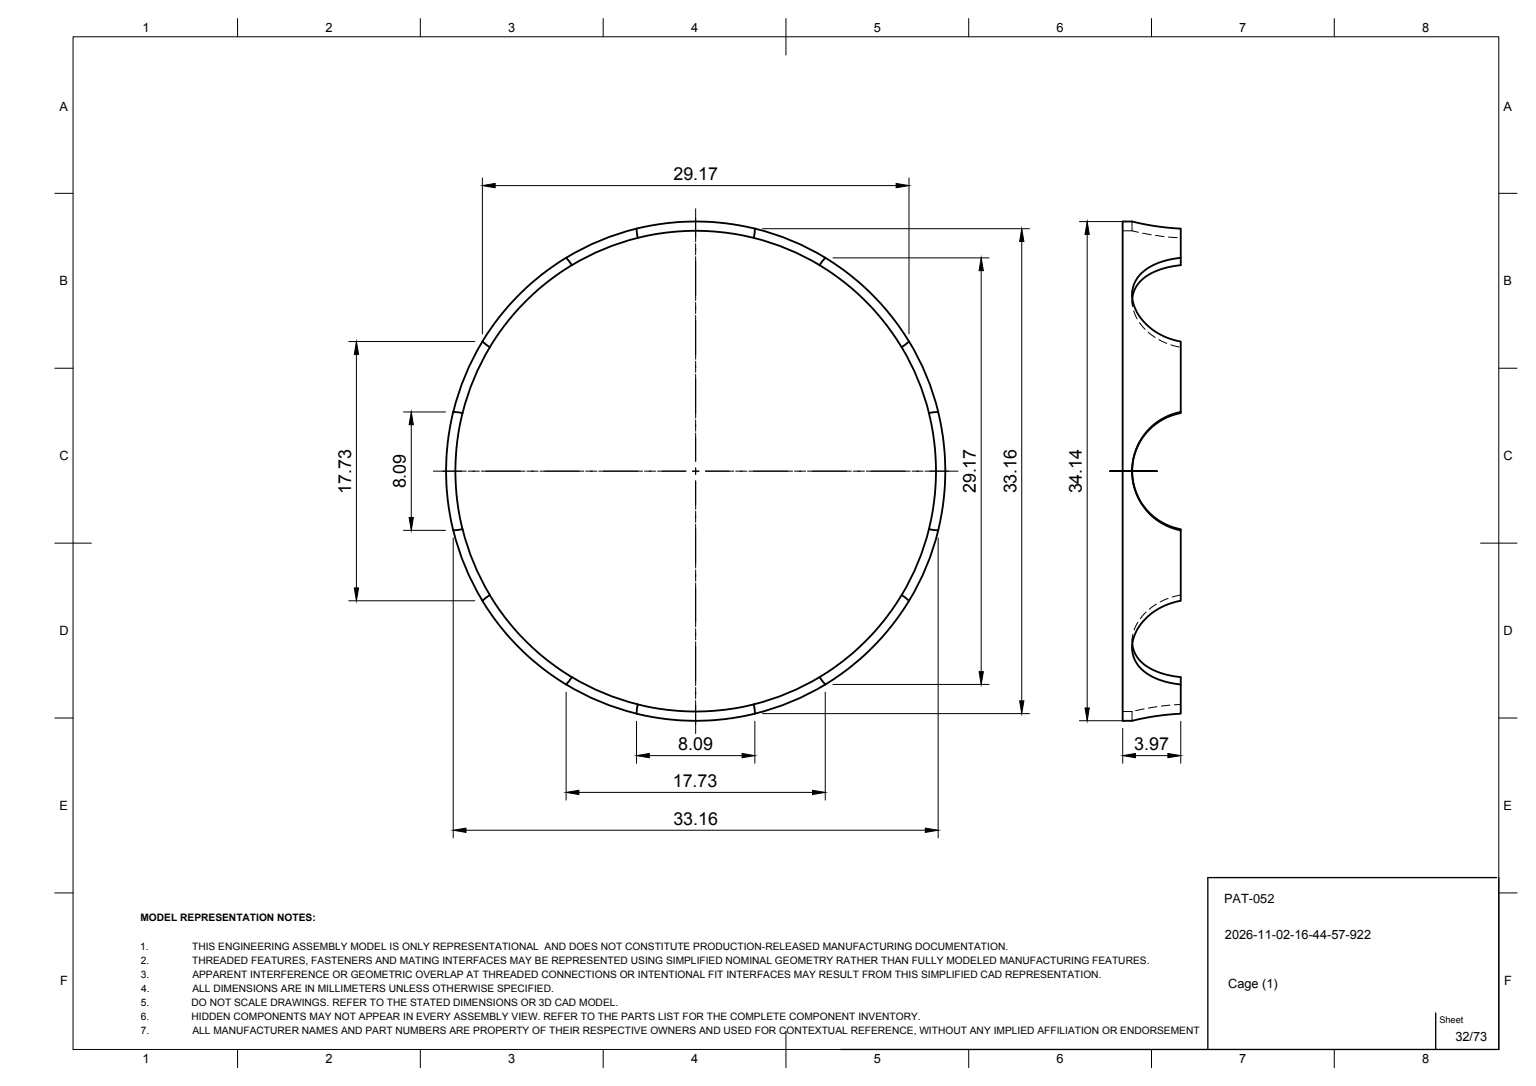
ISO-10303-21;
HEADER;
/* Generated by software containing ST-Developer
 * from STEP Tools, Inc. (www.steptools.com) 
 */

FILE_DESCRIPTION(
/* description */ ('Hand-crank gear train demonstrator'),
/* implementation_level */ '2;1');

FILE_NAME(
/* name */ 'Cage (1).step',
/* time_stamp */ '2026-10-28T03:22:13-07:00',
/* author */ (''),
/* organization */ (''),
/* preprocessor_version */ 'ST-DEVELOPER v20.2',
/* originating_system */ 'Autodesk Translation Framework v15.17.0.0',
/* authorisation */ '');

FILE_SCHEMA (('AUTOMOTIVE_DESIGN { 1 0 10303 214 3 1 1 }'));
ENDSEC;

DATA;
#10=MECHANICAL_DESIGN_GEOMETRIC_PRESENTATION_REPRESENTATION('',(#1222),#62758);
#873=B_SPLINE_CURVE_WITH_KNOTS('',3,(#24613,#24614,#24615,#24616,#24617,
#24618,#24619,#24620,#24621,#24622,#24623,#24624,#24625,#24626,#24627,#24628,
#24629,#24630,#24631,#24632,#24633,#24634),.UNSPECIFIED.,.F.,.F.,(4,2,2,
2,2,2,2,2,2,2,4),(0.0789094028588958,0.210573405340968,0.315860108011452,
0.421146810681936,0.522142632548711,0.623138454415485,0.72413427628226,
0.825130098149035,0.930416800819519,1.03570350349,1.16736750597208),
 .UNSPECIFIED.);
#874=B_SPLINE_CURVE_WITH_KNOTS('',3,(#24638,#24639,#24640,#24641,#24642,
#24643,#24644,#24645,#24646,#24647,#24648,#24649,#24650,#24651,#24652,#24653,
#24654,#24655,#24656,#24657,#24658,#24659),.UNSPECIFIED.,.F.,.F.,(4,2,2,
2,2,2,2,2,2,2,4),(0.0774793363974613,0.142088896491891,0.284177792983782,
0.411119756996526,0.514392970548519,0.617666184100513,0.720939397652506,
0.8242126112045,0.951154575217244,1.09324347170913,1.15785303180356),
 .UNSPECIFIED.);
#875=B_SPLINE_CURVE_WITH_KNOTS('',3,(#24665,#24666,#24667,#24668,#24669,
#24670,#24671,#24672,#24673,#24674,#24675,#24676,#24677,#24678,#24679,#24680,
#24681,#24682,#24683,#24684,#24685,#24686),.UNSPECIFIED.,.F.,.F.,(4,2,2,
2,2,2,2,2,2,2,4),(0.0774793363974613,0.142088896491891,0.284177792983782,
0.411119756996525,0.514392970548519,0.617666184100513,0.720939397652506,
0.8242126112045,0.951154575217243,1.09324347170913,1.15785303180356),
 .UNSPECIFIED.);
#876=B_SPLINE_CURVE_WITH_KNOTS('',3,(#24690,#24691,#24692,#24693,#24694,
#24695,#24696,#24697,#24698,#24699,#24700,#24701,#24702,#24703,#24704,#24705,
#24706,#24707,#24708,#24709,#24710,#24711),.UNSPECIFIED.,.F.,.F.,(4,2,2,
2,2,2,2,2,2,2,4),(0.0774793363974614,0.142088896491891,0.284177792983781,
0.411119756996525,0.514392970548519,0.617666184100512,0.720939397652506,
0.824212611204499,0.951154575217243,1.09324347170913,1.15785303180356),
 .UNSPECIFIED.);
#877=B_SPLINE_CURVE_WITH_KNOTS('',3,(#24715,#24716,#24717,#24718,#24719,
#24720,#24721,#24722,#24723,#24724,#24725,#24726),.UNSPECIFIED.,.F.,.F.,
(4,2,2,2,2,4),(0.0774793363974613,0.142088896491891,0.284177792983781,0.411119756996525,
0.514392970548519,0.617666184100512),.UNSPECIFIED.);
#878=B_SPLINE_CURVE_WITH_KNOTS('',3,(#24731,#24732,#24733,#24734,#24735,
#24736,#24737,#24738,#24739,#24740,#24741,#24742),.UNSPECIFIED.,.F.,.F.,
(4,2,2,2,2,4),(0.617666184100512,0.720939397652506,0.824212611204499,0.951154575217243,
1.09324347170913,1.15785303180356),.UNSPECIFIED.);
#879=B_SPLINE_CURVE_WITH_KNOTS('',3,(#24746,#24747,#24748,#24749,#24750,
#24751,#24752,#24753,#24754,#24755,#24756,#24757,#24758,#24759,#24760,#24761,
#24762,#24763,#24764,#24765,#24766,#24767),.UNSPECIFIED.,.F.,.F.,(4,2,2,
2,2,2,2,2,2,2,4),(0.0774793363974613,0.142088896491891,0.284177792983782,
0.411119756996526,0.514392970548519,0.617666184100513,0.720939397652507,
0.8242126112045,0.951154575217245,1.09324347170914,1.15785303180356),
 .UNSPECIFIED.);
#880=B_SPLINE_CURVE_WITH_KNOTS('',3,(#24771,#24772,#24773,#24774,#24775,
#24776,#24777,#24778,#24779,#24780,#24781,#24782,#24783,#24784,#24785,#24786,
#24787,#24788,#24789,#24790,#24791,#24792),.UNSPECIFIED.,.F.,.F.,(4,2,2,
2,2,2,2,2,2,2,4),(0.0774793363974613,0.142088896491891,0.284177792983782,
0.411119756996526,0.514392970548519,0.617666184100513,0.720939397652506,
0.824212611204499,0.951154575217243,1.09324347170913,1.15785303180356),
 .UNSPECIFIED.);
#881=B_SPLINE_CURVE_WITH_KNOTS('',3,(#24796,#24797,#24798,#24799,#24800,
#24801,#24802,#24803,#24804,#24805,#24806,#24807,#24808,#24809,#24810,#24811,
#24812,#24813,#24814,#24815,#24816,#24817),.UNSPECIFIED.,.F.,.F.,(4,2,2,
2,2,2,2,2,2,2,4),(0.0774793363974613,0.142088896491891,0.284177792983782,
0.411119756996526,0.514392970548519,0.617666184100513,0.720939397652506,
0.8242126112045,0.951154575217244,1.09324347170913,1.15785303180356),
 .UNSPECIFIED.);
#882=B_SPLINE_CURVE_WITH_KNOTS('',3,(#24821,#24822,#24823,#24824,#24825,
#24826,#24827,#24828,#24829,#24830,#24831,#24832,#24833,#24834,#24835,#24836,
#24837,#24838,#24839,#24840,#24841,#24842),.UNSPECIFIED.,.F.,.F.,(4,2,2,
2,2,2,2,2,2,2,4),(0.0774793363974613,0.142088896491891,0.284177792983782,
0.411119756996526,0.514392970548519,0.617666184100513,0.720939397652506,
0.8242126112045,0.951154575217243,1.09324347170913,1.15785303180356),
 .UNSPECIFIED.);
#883=B_SPLINE_CURVE_WITH_KNOTS('',3,(#24850,#24851,#24852,#24853,#24854,
#24855,#24856,#24857,#24858,#24859,#24860,#24861,#24862,#24863,#24864,#24865,
#24866,#24867,#24868,#24869,#24870,#24871),.UNSPECIFIED.,.F.,.F.,(4,2,2,
2,2,2,2,2,2,2,4),(0.0789094028588958,0.210573405340968,0.315860108011452,
0.421146810681936,0.522142632548711,0.623138454415485,0.72413427628226,
0.825130098149035,0.930416800819519,1.03570350349,1.16736750597208),
 .UNSPECIFIED.);
#884=B_SPLINE_CURVE_WITH_KNOTS('',3,(#24879,#24880,#24881,#24882,#24883,
#24884,#24885,#24886,#24887,#24888,#24889,#24890,#24891,#24892,#24893,#24894,
#24895,#24896,#24897,#24898,#24899,#24900),.UNSPECIFIED.,.F.,.F.,(4,2,2,
2,2,2,2,2,2,2,4),(0.0789094028588958,0.210573405340969,0.315860108011453,
0.421146810681937,0.522142632548712,0.623138454415486,0.724134276282261,
0.825130098149035,0.930416800819519,1.03570350349,1.16736750597208),
 .UNSPECIFIED.);
#885=B_SPLINE_CURVE_WITH_KNOTS('',3,(#24909,#24910,#24911,#24912,#24913,
#24914,#24915,#24916,#24917,#24918,#24919,#24920),.UNSPECIFIED.,.F.,.F.,
(4,2,2,2,2,4),(0.0789094028588958,0.210573405340968,0.315860108011452,0.421146810681937,
0.522142632548711,0.623138454415486),.UNSPECIFIED.);
#886=B_SPLINE_CURVE_WITH_KNOTS('',3,(#24922,#24923,#24924,#24925,#24926,
#24927,#24928,#24929,#24930,#24931,#24932,#24933),.UNSPECIFIED.,.F.,.F.,
(4,2,2,2,2,4),(0.623138454415486,0.72413427628226,0.825130098149035,0.930416800819519,
1.03570350349,1.16736750597208),.UNSPECIFIED.);
#887=B_SPLINE_CURVE_WITH_KNOTS('',3,(#24940,#24941,#24942,#24943,#24944,
#24945,#24946,#24947,#24948,#24949,#24950,#24951,#24952,#24953,#24954,#24955,
#24956,#24957,#24958,#24959,#24960,#24961),.UNSPECIFIED.,.F.,.F.,(4,2,2,
2,2,2,2,2,2,2,4),(0.0789094028588958,0.210573405340968,0.315860108011452,
0.421146810681936,0.522142632548711,0.623138454415486,0.72413427628226,
0.825130098149035,0.930416800819519,1.03570350349,1.16736750597208),
 .UNSPECIFIED.);
#888=B_SPLINE_CURVE_WITH_KNOTS('',3,(#24969,#24970,#24971,#24972,#24973,
#24974,#24975,#24976,#24977,#24978,#24979,#24980,#24981,#24982,#24983,#24984,
#24985,#24986,#24987,#24988,#24989,#24990),.UNSPECIFIED.,.F.,.F.,(4,2,2,
2,2,2,2,2,2,2,4),(0.0789094028588957,0.210573405340968,0.315860108011452,
0.421146810681936,0.522142632548711,0.623138454415485,0.72413427628226,
0.825130098149035,0.930416800819519,1.03570350349,1.16736750597207),
 .UNSPECIFIED.);
#889=B_SPLINE_CURVE_WITH_KNOTS('',3,(#24998,#24999,#25000,#25001,#25002,
#25003,#25004,#25005,#25006,#25007,#25008,#25009,#25010,#25011,#25012,#25013,
#25014,#25015,#25016,#25017,#25018,#25019),.UNSPECIFIED.,.F.,.F.,(4,2,2,
2,2,2,2,2,2,2,4),(0.0789094028588958,0.210573405340968,0.315860108011452,
0.421146810681936,0.522142632548711,0.623138454415486,0.72413427628226,
0.825130098149035,0.930416800819519,1.03570350349,1.16736750597208),
 .UNSPECIFIED.);
#890=B_SPLINE_CURVE_WITH_KNOTS('',3,(#25028,#25029,#25030,#25031,#25032,
#25033,#25034,#25035,#25036,#25037,#25038,#25039,#25040,#25041,#25042,#25043,
#25044,#25045,#25046,#25047,#25048,#25049),.UNSPECIFIED.,.F.,.F.,(4,2,2,
2,2,2,2,2,2,2,4),(0.0789094028588958,0.210573405340968,0.315860108011452,
0.421146810681936,0.522142632548711,0.623138454415485,0.72413427628226,
0.825130098149035,0.930416800819519,1.03570350349,1.16736750597208),
 .UNSPECIFIED.);
#1013=SPHERICAL_SURFACE('',#17671,0.412776);
#1014=SPHERICAL_SURFACE('',#17687,0.412776);
#1015=SPHERICAL_SURFACE('',#17692,0.412776);
#1016=SPHERICAL_SURFACE('',#17697,0.412776);
#1017=SPHERICAL_SURFACE('',#17702,0.412776);
#1018=SPHERICAL_SURFACE('',#17707,0.412776);
#1019=SPHERICAL_SURFACE('',#17712,0.412776);
#1020=SPHERICAL_SURFACE('',#17720,0.412776);
#1080=SHAPE_REPRESENTATION_RELATIONSHIP('SRR','None',#63054,#1144);
#1144=ADVANCED_BREP_SHAPE_REPRESENTATION('',(#1300),#62708);
#1222=STYLED_ITEM('',(#63462),#1300);
#1300=MANIFOLD_SOLID_BREP('Continuous crown cage',#16403);
#1500=FACE_BOUND('',#3445,.T.);
#1702=PLANE('',#17684);
#1703=PLANE('',#17689);
#1704=PLANE('',#17694);
#1705=PLANE('',#17699);
#1706=PLANE('',#17704);
#1707=PLANE('',#17709);
#1708=PLANE('',#17718);
#1709=PLANE('',#17722);
#1710=PLANE('',#17723);
#2333=FACE_OUTER_BOUND('',#3427,.T.);
#2334=FACE_OUTER_BOUND('',#3428,.T.);
#2335=FACE_OUTER_BOUND('',#3429,.T.);
#2336=FACE_OUTER_BOUND('',#3430,.T.);
#2337=FACE_OUTER_BOUND('',#3431,.T.);
#2338=FACE_OUTER_BOUND('',#3432,.T.);
#2339=FACE_OUTER_BOUND('',#3433,.T.);
#2340=FACE_OUTER_BOUND('',#3434,.T.);
#2341=FACE_OUTER_BOUND('',#3435,.T.);
#2342=FACE_OUTER_BOUND('',#3436,.T.);
#2343=FACE_OUTER_BOUND('',#3437,.T.);
#2344=FACE_OUTER_BOUND('',#3438,.T.);
#2345=FACE_OUTER_BOUND('',#3439,.T.);
#2346=FACE_OUTER_BOUND('',#3440,.T.);
#2347=FACE_OUTER_BOUND('',#3441,.T.);
#2348=FACE_OUTER_BOUND('',#3442,.T.);
#2349=FACE_OUTER_BOUND('',#3443,.T.);
#2350=FACE_OUTER_BOUND('',#3444,.T.);
#2351=FACE_OUTER_BOUND('',#3446,.T.);
#3427=EDGE_LOOP('',(#11737,#11738,#11739,#11740));
#3428=EDGE_LOOP('',(#11741,#11742,#11743,#11744,#11745,#11746,#11747,#11748,
#11749,#11750,#11751,#11752,#11753,#11754,#11755,#11756,#11757,#11758,#11759,
#11760));
#3429=EDGE_LOOP('',(#11761,#11762,#11763,#11764));
#3430=EDGE_LOOP('',(#11765,#11766,#11767,#11768));
#3431=EDGE_LOOP('',(#11769,#11770,#11771,#11772));
#3432=EDGE_LOOP('',(#11773,#11774,#11775,#11776));
#3433=EDGE_LOOP('',(#11777,#11778,#11779,#11780));
#3434=EDGE_LOOP('',(#11781,#11782,#11783,#11784,#11785,#11786));
#3435=EDGE_LOOP('',(#11787,#11788,#11789,#11790));
#3436=EDGE_LOOP('',(#11791,#11792,#11793,#11794));
#3437=EDGE_LOOP('',(#11795,#11796,#11797,#11798));
#3438=EDGE_LOOP('',(#11799,#11800,#11801,#11802));
#3439=EDGE_LOOP('',(#11803,#11804,#11805,#11806));
#3440=EDGE_LOOP('',(#11807,#11808,#11809,#11810));
#3441=EDGE_LOOP('',(#11811,#11812,#11813,#11814,#11815,#11816,#11817,#11818,
#11819,#11820,#11821,#11822,#11823,#11824,#11825,#11826,#11827,#11828,#11829,
#11830));
#3442=EDGE_LOOP('',(#11831,#11832,#11833,#11834));
#3443=EDGE_LOOP('',(#11835,#11836,#11837,#11838));
#3444=EDGE_LOOP('',(#11839));
#3445=EDGE_LOOP('',(#11840));
#3446=EDGE_LOOP('',(#11841,#11842,#11843,#11844));
#4449=LINE('',#24728,#5581);
#4450=LINE('',#25024,#5582);
#5581=VECTOR('',#20034,1.706752);
#5582=VECTOR('',#20111,1.643248);
#6824=CIRCLE('',#17672,0.405071403305639);
#6825=CIRCLE('',#17673,0.405071403305639);
#6826=CIRCLE('',#17675,1.706752);
#6827=CIRCLE('',#17676,1.706752);
#6828=CIRCLE('',#17677,1.706752);
#6829=CIRCLE('',#17678,1.706752);
#6830=CIRCLE('',#17679,1.706752);
#6831=CIRCLE('',#17680,1.706752);
#6832=CIRCLE('',#17681,1.706752);
#6833=CIRCLE('',#17682,1.706752);
#6834=CIRCLE('',#17683,1.706752);
#6835=CIRCLE('',#17685,1.643248);
#6836=CIRCLE('',#17686,0.405071403305639);
#6837=CIRCLE('',#17688,0.405071403305639);
#6838=CIRCLE('',#17690,1.643248);
#6839=CIRCLE('',#17691,0.405071403305639);
#6840=CIRCLE('',#17693,0.405071403305639);
#6841=CIRCLE('',#17695,1.643248);
#6842=CIRCLE('',#17696,0.405071403305639);
#6843=CIRCLE('',#17698,0.405071403305639);
#6844=CIRCLE('',#17700,1.643248);
#6845=CIRCLE('',#17701,0.405071403305639);
#6846=CIRCLE('',#17703,0.405071403305639);
#6847=CIRCLE('',#17705,1.643248);
#6848=CIRCLE('',#17706,0.405071403305639);
#6849=CIRCLE('',#17708,0.405071403305639);
#6850=CIRCLE('',#17710,1.643248);
#6851=CIRCLE('',#17711,0.405071403305639);
#6852=CIRCLE('',#17713,0.405071403305639);
#6853=CIRCLE('',#17715,1.643248);
#6854=CIRCLE('',#17716,1.643248);
#6855=CIRCLE('',#17717,1.643248);
#6856=CIRCLE('',#17719,0.405071403305639);
#6857=CIRCLE('',#17721,0.405071403305639);
#7529=VERTEX_POINT('',#24611);
#7530=VERTEX_POINT('',#24612);
#7531=VERTEX_POINT('',#24635);
#7532=VERTEX_POINT('',#24637);
#7533=VERTEX_POINT('',#24662);
#7534=VERTEX_POINT('',#24664);
#7535=VERTEX_POINT('',#24687);
#7536=VERTEX_POINT('',#24689);
#7537=VERTEX_POINT('',#24712);
#7538=VERTEX_POINT('',#24714);
#7539=VERTEX_POINT('',#24727);
#7540=VERTEX_POINT('',#24730);
#7541=VERTEX_POINT('',#24743);
#7542=VERTEX_POINT('',#24745);
#7543=VERTEX_POINT('',#24768);
#7544=VERTEX_POINT('',#24770);
#7545=VERTEX_POINT('',#24793);
#7546=VERTEX_POINT('',#24795);
#7547=VERTEX_POINT('',#24818);
#7548=VERTEX_POINT('',#24820);
#7549=VERTEX_POINT('',#24845);
#7550=VERTEX_POINT('',#24849);
#7551=VERTEX_POINT('',#24874);
#7552=VERTEX_POINT('',#24878);
#7553=VERTEX_POINT('',#24903);
#7554=VERTEX_POINT('',#24907);
#7555=VERTEX_POINT('',#24908);
#7556=VERTEX_POINT('',#24935);
#7557=VERTEX_POINT('',#24939);
#7558=VERTEX_POINT('',#24964);
#7559=VERTEX_POINT('',#24968);
#7560=VERTEX_POINT('',#24993);
#7561=VERTEX_POINT('',#24997);
#7562=VERTEX_POINT('',#25022);
#7563=VERTEX_POINT('',#25025);
#7564=VERTEX_POINT('',#25027);
#9120=EDGE_CURVE('',#7529,#7530,#873,.T.);
#9121=EDGE_CURVE('',#7531,#7529,#6824,.T.);
#9122=EDGE_CURVE('',#7532,#7531,#874,.T.);
#9123=EDGE_CURVE('',#7530,#7532,#6825,.T.);
#9124=EDGE_CURVE('',#7533,#7531,#6826,.T.);
#9125=EDGE_CURVE('',#7533,#7534,#875,.T.);
#9126=EDGE_CURVE('',#7535,#7534,#6827,.T.);
#9127=EDGE_CURVE('',#7535,#7536,#876,.T.);
#9128=EDGE_CURVE('',#7537,#7536,#6828,.T.);
#9129=EDGE_CURVE('',#7537,#7538,#877,.T.);
#9130=EDGE_CURVE('',#7538,#7539,#4449,.T.);
#9131=EDGE_CURVE('',#7539,#7539,#6829,.T.);
#9132=EDGE_CURVE('',#7538,#7540,#878,.T.);
#9133=EDGE_CURVE('',#7541,#7540,#6830,.T.);
#9134=EDGE_CURVE('',#7541,#7542,#879,.T.);
#9135=EDGE_CURVE('',#7543,#7542,#6831,.T.);
#9136=EDGE_CURVE('',#7543,#7544,#880,.T.);
#9137=EDGE_CURVE('',#7545,#7544,#6832,.T.);
#9138=EDGE_CURVE('',#7545,#7546,#881,.T.);
#9139=EDGE_CURVE('',#7547,#7546,#6833,.T.);
#9140=EDGE_CURVE('',#7547,#7548,#882,.T.);
#9141=EDGE_CURVE('',#7532,#7548,#6834,.T.);
#9142=EDGE_CURVE('',#7529,#7549,#6835,.T.);
#9143=EDGE_CURVE('',#7549,#7533,#6836,.T.);
#9144=EDGE_CURVE('',#7550,#7549,#883,.T.);
#9145=EDGE_CURVE('',#7534,#7550,#6837,.T.);
#9146=EDGE_CURVE('',#7550,#7551,#6838,.T.);
#9147=EDGE_CURVE('',#7551,#7535,#6839,.T.);
#9148=EDGE_CURVE('',#7552,#7551,#884,.T.);
#9149=EDGE_CURVE('',#7536,#7552,#6840,.T.);
#9150=EDGE_CURVE('',#7552,#7553,#6841,.T.);
#9151=EDGE_CURVE('',#7553,#7537,#6842,.T.);
#9152=EDGE_CURVE('',#7554,#7555,#885,.T.);
#9153=EDGE_CURVE('',#7540,#7554,#6843,.T.);
#9154=EDGE_CURVE('',#7555,#7553,#886,.T.);
#9155=EDGE_CURVE('',#7554,#7556,#6844,.T.);
#9156=EDGE_CURVE('',#7556,#7541,#6845,.T.);
#9157=EDGE_CURVE('',#7557,#7556,#887,.T.);
#9158=EDGE_CURVE('',#7542,#7557,#6846,.T.);
#9159=EDGE_CURVE('',#7557,#7558,#6847,.T.);
#9160=EDGE_CURVE('',#7558,#7543,#6848,.T.);
#9161=EDGE_CURVE('',#7559,#7558,#888,.T.);
#9162=EDGE_CURVE('',#7544,#7559,#6849,.T.);
#9163=EDGE_CURVE('',#7559,#7560,#6850,.T.);
#9164=EDGE_CURVE('',#7560,#7545,#6851,.T.);
#9165=EDGE_CURVE('',#7561,#7560,#889,.T.);
#9166=EDGE_CURVE('',#7546,#7561,#6852,.T.);
#9167=EDGE_CURVE('',#7562,#7562,#6853,.T.);
#9168=EDGE_CURVE('',#7562,#7555,#4450,.T.);
#9169=EDGE_CURVE('',#7563,#7530,#6854,.T.);
#9170=EDGE_CURVE('',#7563,#7564,#890,.T.);
#9171=EDGE_CURVE('',#7561,#7564,#6855,.T.);
#9172=EDGE_CURVE('',#7548,#7563,#6856,.T.);
#9173=EDGE_CURVE('',#7564,#7547,#6857,.T.);
#11737=ORIENTED_EDGE('',*,*,#9120,.F.);
#11738=ORIENTED_EDGE('',*,*,#9121,.F.);
#11739=ORIENTED_EDGE('',*,*,#9122,.F.);
#11740=ORIENTED_EDGE('',*,*,#9123,.F.);
#11741=ORIENTED_EDGE('',*,*,#9122,.T.);
#11742=ORIENTED_EDGE('',*,*,#9124,.F.);
#11743=ORIENTED_EDGE('',*,*,#9125,.T.);
#11744=ORIENTED_EDGE('',*,*,#9126,.F.);
#11745=ORIENTED_EDGE('',*,*,#9127,.T.);
#11746=ORIENTED_EDGE('',*,*,#9128,.F.);
#11747=ORIENTED_EDGE('',*,*,#9129,.T.);
#11748=ORIENTED_EDGE('',*,*,#9130,.T.);
#11749=ORIENTED_EDGE('',*,*,#9131,.F.);
#11750=ORIENTED_EDGE('',*,*,#9130,.F.);
#11751=ORIENTED_EDGE('',*,*,#9132,.T.);
#11752=ORIENTED_EDGE('',*,*,#9133,.F.);
#11753=ORIENTED_EDGE('',*,*,#9134,.T.);
#11754=ORIENTED_EDGE('',*,*,#9135,.F.);
#11755=ORIENTED_EDGE('',*,*,#9136,.T.);
#11756=ORIENTED_EDGE('',*,*,#9137,.F.);
#11757=ORIENTED_EDGE('',*,*,#9138,.T.);
#11758=ORIENTED_EDGE('',*,*,#9139,.F.);
#11759=ORIENTED_EDGE('',*,*,#9140,.T.);
#11760=ORIENTED_EDGE('',*,*,#9141,.F.);
#11761=ORIENTED_EDGE('',*,*,#9121,.T.);
#11762=ORIENTED_EDGE('',*,*,#9142,.T.);
#11763=ORIENTED_EDGE('',*,*,#9143,.T.);
#11764=ORIENTED_EDGE('',*,*,#9124,.T.);
#11765=ORIENTED_EDGE('',*,*,#9144,.F.);
#11766=ORIENTED_EDGE('',*,*,#9145,.F.);
#11767=ORIENTED_EDGE('',*,*,#9125,.F.);
#11768=ORIENTED_EDGE('',*,*,#9143,.F.);
#11769=ORIENTED_EDGE('',*,*,#9145,.T.);
#11770=ORIENTED_EDGE('',*,*,#9146,.T.);
#11771=ORIENTED_EDGE('',*,*,#9147,.T.);
#11772=ORIENTED_EDGE('',*,*,#9126,.T.);
#11773=ORIENTED_EDGE('',*,*,#9148,.F.);
#11774=ORIENTED_EDGE('',*,*,#9149,.F.);
#11775=ORIENTED_EDGE('',*,*,#9127,.F.);
#11776=ORIENTED_EDGE('',*,*,#9147,.F.);
#11777=ORIENTED_EDGE('',*,*,#9149,.T.);
#11778=ORIENTED_EDGE('',*,*,#9150,.T.);
#11779=ORIENTED_EDGE('',*,*,#9151,.T.);
#11780=ORIENTED_EDGE('',*,*,#9128,.T.);
#11781=ORIENTED_EDGE('',*,*,#9152,.F.);
#11782=ORIENTED_EDGE('',*,*,#9153,.F.);
#11783=ORIENTED_EDGE('',*,*,#9132,.F.);
#11784=ORIENTED_EDGE('',*,*,#9129,.F.);
#11785=ORIENTED_EDGE('',*,*,#9151,.F.);
#11786=ORIENTED_EDGE('',*,*,#9154,.F.);
#11787=ORIENTED_EDGE('',*,*,#9153,.T.);
#11788=ORIENTED_EDGE('',*,*,#9155,.T.);
#11789=ORIENTED_EDGE('',*,*,#9156,.T.);
#11790=ORIENTED_EDGE('',*,*,#9133,.T.);
#11791=ORIENTED_EDGE('',*,*,#9157,.F.);
#11792=ORIENTED_EDGE('',*,*,#9158,.F.);
#11793=ORIENTED_EDGE('',*,*,#9134,.F.);
#11794=ORIENTED_EDGE('',*,*,#9156,.F.);
#11795=ORIENTED_EDGE('',*,*,#9158,.T.);
#11796=ORIENTED_EDGE('',*,*,#9159,.T.);
#11797=ORIENTED_EDGE('',*,*,#9160,.T.);
#11798=ORIENTED_EDGE('',*,*,#9135,.T.);
#11799=ORIENTED_EDGE('',*,*,#9161,.F.);
#11800=ORIENTED_EDGE('',*,*,#9162,.F.);
#11801=ORIENTED_EDGE('',*,*,#9136,.F.);
#11802=ORIENTED_EDGE('',*,*,#9160,.F.);
#11803=ORIENTED_EDGE('',*,*,#9162,.T.);
#11804=ORIENTED_EDGE('',*,*,#9163,.T.);
#11805=ORIENTED_EDGE('',*,*,#9164,.T.);
#11806=ORIENTED_EDGE('',*,*,#9137,.T.);
#11807=ORIENTED_EDGE('',*,*,#9138,.F.);
#11808=ORIENTED_EDGE('',*,*,#9164,.F.);
#11809=ORIENTED_EDGE('',*,*,#9165,.F.);
#11810=ORIENTED_EDGE('',*,*,#9166,.F.);
#11811=ORIENTED_EDGE('',*,*,#9167,.F.);
#11812=ORIENTED_EDGE('',*,*,#9168,.T.);
#11813=ORIENTED_EDGE('',*,*,#9154,.T.);
#11814=ORIENTED_EDGE('',*,*,#9150,.F.);
#11815=ORIENTED_EDGE('',*,*,#9148,.T.);
#11816=ORIENTED_EDGE('',*,*,#9146,.F.);
#11817=ORIENTED_EDGE('',*,*,#9144,.T.);
#11818=ORIENTED_EDGE('',*,*,#9142,.F.);
#11819=ORIENTED_EDGE('',*,*,#9120,.T.);
#11820=ORIENTED_EDGE('',*,*,#9169,.F.);
#11821=ORIENTED_EDGE('',*,*,#9170,.T.);
#11822=ORIENTED_EDGE('',*,*,#9171,.F.);
#11823=ORIENTED_EDGE('',*,*,#9165,.T.);
#11824=ORIENTED_EDGE('',*,*,#9163,.F.);
#11825=ORIENTED_EDGE('',*,*,#9161,.T.);
#11826=ORIENTED_EDGE('',*,*,#9159,.F.);
#11827=ORIENTED_EDGE('',*,*,#9157,.T.);
#11828=ORIENTED_EDGE('',*,*,#9155,.F.);
#11829=ORIENTED_EDGE('',*,*,#9152,.T.);
#11830=ORIENTED_EDGE('',*,*,#9168,.F.);
#11831=ORIENTED_EDGE('',*,*,#9123,.T.);
#11832=ORIENTED_EDGE('',*,*,#9141,.T.);
#11833=ORIENTED_EDGE('',*,*,#9172,.T.);
#11834=ORIENTED_EDGE('',*,*,#9169,.T.);
#11835=ORIENTED_EDGE('',*,*,#9140,.F.);
#11836=ORIENTED_EDGE('',*,*,#9173,.F.);
#11837=ORIENTED_EDGE('',*,*,#9170,.F.);
#11838=ORIENTED_EDGE('',*,*,#9172,.F.);
#11839=ORIENTED_EDGE('',*,*,#9131,.T.);
#11840=ORIENTED_EDGE('',*,*,#9167,.T.);
#11841=ORIENTED_EDGE('',*,*,#9166,.T.);
#11842=ORIENTED_EDGE('',*,*,#9171,.T.);
#11843=ORIENTED_EDGE('',*,*,#9173,.T.);
#11844=ORIENTED_EDGE('',*,*,#9139,.T.);
#15271=CYLINDRICAL_SURFACE('',#17674,1.706752);
#15272=CYLINDRICAL_SURFACE('',#17714,1.643248);
#15643=ADVANCED_FACE('',(#2333),#1013,.F.);
#15644=ADVANCED_FACE('',(#2334),#15271,.T.);
#15645=ADVANCED_FACE('',(#2335),#1702,.T.);
#15646=ADVANCED_FACE('',(#2336),#1014,.F.);
#15647=ADVANCED_FACE('',(#2337),#1703,.T.);
#15648=ADVANCED_FACE('',(#2338),#1015,.F.);
#15649=ADVANCED_FACE('',(#2339),#1704,.T.);
#15650=ADVANCED_FACE('',(#2340),#1016,.F.);
#15651=ADVANCED_FACE('',(#2341),#1705,.T.);
#15652=ADVANCED_FACE('',(#2342),#1017,.F.);
#15653=ADVANCED_FACE('',(#2343),#1706,.T.);
#15654=ADVANCED_FACE('',(#2344),#1018,.F.);
#15655=ADVANCED_FACE('',(#2345),#1707,.T.);
#15656=ADVANCED_FACE('',(#2346),#1019,.F.);
#15657=ADVANCED_FACE('',(#2347),#15272,.F.);
#15658=ADVANCED_FACE('',(#2348),#1708,.T.);
#15659=ADVANCED_FACE('',(#2349),#1020,.F.);
#15660=ADVANCED_FACE('',(#2350,#1500),#1709,.T.);
#15661=ADVANCED_FACE('',(#2351),#1710,.T.);
#16403=CLOSED_SHELL('',(#15643,#15644,#15645,#15646,#15647,#15648,#15649,
#15650,#15651,#15652,#15653,#15654,#15655,#15656,#15657,#15658,#15659,#15660,
#15661));
#17670=AXIS2_PLACEMENT_3D('',#24609,#20018,#20019);
#17671=AXIS2_PLACEMENT_3D('',#24610,#20020,#20021);
#17672=AXIS2_PLACEMENT_3D('',#24636,#20022,#20023);
#17673=AXIS2_PLACEMENT_3D('',#24660,#20024,#20025);
#17674=AXIS2_PLACEMENT_3D('',#24661,#20026,#20027);
#17675=AXIS2_PLACEMENT_3D('',#24663,#20028,#20029);
#17676=AXIS2_PLACEMENT_3D('',#24688,#20030,#20031);
#17677=AXIS2_PLACEMENT_3D('',#24713,#20032,#20033);
#17678=AXIS2_PLACEMENT_3D('',#24729,#20035,#20036);
#17679=AXIS2_PLACEMENT_3D('',#24744,#20037,#20038);
#17680=AXIS2_PLACEMENT_3D('',#24769,#20039,#20040);
#17681=AXIS2_PLACEMENT_3D('',#24794,#20041,#20042);
#17682=AXIS2_PLACEMENT_3D('',#24819,#20043,#20044);
#17683=AXIS2_PLACEMENT_3D('',#24843,#20045,#20046);
#17684=AXIS2_PLACEMENT_3D('',#24844,#20047,#20048);
#17685=AXIS2_PLACEMENT_3D('',#24846,#20049,#20050);
#17686=AXIS2_PLACEMENT_3D('',#24847,#20051,#20052);
#17687=AXIS2_PLACEMENT_3D('',#24848,#20053,#20054);
#17688=AXIS2_PLACEMENT_3D('',#24872,#20055,#20056);
#17689=AXIS2_PLACEMENT_3D('',#24873,#20057,#20058);
#17690=AXIS2_PLACEMENT_3D('',#24875,#20059,#20060);
#17691=AXIS2_PLACEMENT_3D('',#24876,#20061,#20062);
#17692=AXIS2_PLACEMENT_3D('',#24877,#20063,#20064);
#17693=AXIS2_PLACEMENT_3D('',#24901,#20065,#20066);
#17694=AXIS2_PLACEMENT_3D('',#24902,#20067,#20068);
#17695=AXIS2_PLACEMENT_3D('',#24904,#20069,#20070);
#17696=AXIS2_PLACEMENT_3D('',#24905,#20071,#20072);
#17697=AXIS2_PLACEMENT_3D('',#24906,#20073,#20074);
#17698=AXIS2_PLACEMENT_3D('',#24921,#20075,#20076);
#17699=AXIS2_PLACEMENT_3D('',#24934,#20077,#20078);
#17700=AXIS2_PLACEMENT_3D('',#24936,#20079,#20080);
#17701=AXIS2_PLACEMENT_3D('',#24937,#20081,#20082);
#17702=AXIS2_PLACEMENT_3D('',#24938,#20083,#20084);
#17703=AXIS2_PLACEMENT_3D('',#24962,#20085,#20086);
#17704=AXIS2_PLACEMENT_3D('',#24963,#20087,#20088);
#17705=AXIS2_PLACEMENT_3D('',#24965,#20089,#20090);
#17706=AXIS2_PLACEMENT_3D('',#24966,#20091,#20092);
#17707=AXIS2_PLACEMENT_3D('',#24967,#20093,#20094);
#17708=AXIS2_PLACEMENT_3D('',#24991,#20095,#20096);
#17709=AXIS2_PLACEMENT_3D('',#24992,#20097,#20098);
#17710=AXIS2_PLACEMENT_3D('',#24994,#20099,#20100);
#17711=AXIS2_PLACEMENT_3D('',#24995,#20101,#20102);
#17712=AXIS2_PLACEMENT_3D('',#24996,#20103,#20104);
#17713=AXIS2_PLACEMENT_3D('',#25020,#20105,#20106);
#17714=AXIS2_PLACEMENT_3D('',#25021,#20107,#20108);
#17715=AXIS2_PLACEMENT_3D('',#25023,#20109,#20110);
#17716=AXIS2_PLACEMENT_3D('',#25026,#20112,#20113);
#17717=AXIS2_PLACEMENT_3D('',#25050,#20114,#20115);
#17718=AXIS2_PLACEMENT_3D('',#25051,#20116,#20117);
#17719=AXIS2_PLACEMENT_3D('',#25052,#20118,#20119);
#17720=AXIS2_PLACEMENT_3D('',#25053,#20120,#20121);
#17721=AXIS2_PLACEMENT_3D('',#25054,#20122,#20123);
#17722=AXIS2_PLACEMENT_3D('',#25055,#20124,#20125);
#17723=AXIS2_PLACEMENT_3D('',#25056,#20126,#20127);
#20018=DIRECTION('axis',(0.,0.,1.));
#20019=DIRECTION('refdir',(1.,0.,0.));
#20020=DIRECTION('center_axis',(0.,0.,1.));
#20021=DIRECTION('ref_axis',(1.,0.,0.));
#20022=DIRECTION('center_axis',(0.,-1.,0.));
#20023=DIRECTION('ref_axis',(0.,0.,-1.));
#20024=DIRECTION('center_axis',(0.,-1.,0.));
#20025=DIRECTION('ref_axis',(0.,0.,-1.));
#20026=DIRECTION('center_axis',(0.,1.,0.));
#20027=DIRECTION('ref_axis',(1.,0.,0.));
#20028=DIRECTION('center_axis',(0.,1.,0.));
#20029=DIRECTION('ref_axis',(1.,0.,0.));
#20030=DIRECTION('center_axis',(0.,1.,0.));
#20031=DIRECTION('ref_axis',(1.,0.,0.));
#20032=DIRECTION('center_axis',(0.,1.,0.));
#20033=DIRECTION('ref_axis',(1.,0.,0.));
#20034=DIRECTION('',(0.,-1.,0.));
#20035=DIRECTION('center_axis',(0.,-1.,0.));
#20036=DIRECTION('ref_axis',(1.,0.,0.));
#20037=DIRECTION('center_axis',(0.,1.,0.));
#20038=DIRECTION('ref_axis',(1.,0.,0.));
#20039=DIRECTION('center_axis',(0.,1.,0.));
#20040=DIRECTION('ref_axis',(1.,0.,0.));
#20041=DIRECTION('center_axis',(0.,1.,0.));
#20042=DIRECTION('ref_axis',(1.,0.,0.));
#20043=DIRECTION('center_axis',(0.,1.,0.));
#20044=DIRECTION('ref_axis',(1.,0.,0.));
#20045=DIRECTION('center_axis',(0.,1.,0.));
#20046=DIRECTION('ref_axis',(1.,0.,0.));
#20047=DIRECTION('center_axis',(0.,1.,0.));
#20048=DIRECTION('ref_axis',(1.,0.,0.));
#20049=DIRECTION('center_axis',(0.,-1.,0.));
#20050=DIRECTION('ref_axis',(1.,0.,0.));
#20051=DIRECTION('center_axis',(0.,-1.,0.));
#20052=DIRECTION('ref_axis',(0.,0.,-1.));
#20053=DIRECTION('center_axis',(6.12323399573677E-17,0.,1.));
#20054=DIRECTION('ref_axis',(1.,0.,0.));
#20055=DIRECTION('center_axis',(0.,-1.,0.));
#20056=DIRECTION('ref_axis',(0.,0.,-1.));
#20057=DIRECTION('center_axis',(0.,1.,0.));
#20058=DIRECTION('ref_axis',(1.,0.,0.));
#20059=DIRECTION('center_axis',(0.,-1.,0.));
#20060=DIRECTION('ref_axis',(1.,0.,0.));
#20061=DIRECTION('center_axis',(0.,-1.,0.));
#20062=DIRECTION('ref_axis',(0.,0.,-1.));
#20063=DIRECTION('center_axis',(0.,0.,1.));
#20064=DIRECTION('ref_axis',(1.,0.,0.));
#20065=DIRECTION('center_axis',(0.,-1.,0.));
#20066=DIRECTION('ref_axis',(0.,0.,-1.));
#20067=DIRECTION('center_axis',(0.,1.,0.));
#20068=DIRECTION('ref_axis',(1.,0.,0.));
#20069=DIRECTION('center_axis',(0.,-1.,0.));
#20070=DIRECTION('ref_axis',(1.,0.,0.));
#20071=DIRECTION('center_axis',(0.,-1.,0.));
#20072=DIRECTION('ref_axis',(0.,0.,-1.));
#20073=DIRECTION('center_axis',(0.,0.,1.));
#20074=DIRECTION('ref_axis',(1.,0.,0.));
#20075=DIRECTION('center_axis',(0.,-1.,0.));
#20076=DIRECTION('ref_axis',(0.,0.,-1.));
#20077=DIRECTION('center_axis',(0.,1.,0.));
#20078=DIRECTION('ref_axis',(1.,0.,0.));
#20079=DIRECTION('center_axis',(0.,-1.,0.));
#20080=DIRECTION('ref_axis',(1.,0.,0.));
#20081=DIRECTION('center_axis',(0.,-1.,0.));
#20082=DIRECTION('ref_axis',(0.,0.,-1.));
#20083=DIRECTION('center_axis',(0.,0.,1.));
#20084=DIRECTION('ref_axis',(1.,0.,0.));
#20085=DIRECTION('center_axis',(0.,-1.,0.));
#20086=DIRECTION('ref_axis',(0.,0.,-1.));
#20087=DIRECTION('center_axis',(0.,1.,0.));
#20088=DIRECTION('ref_axis',(1.,0.,0.));
#20089=DIRECTION('center_axis',(0.,-1.,0.));
#20090=DIRECTION('ref_axis',(1.,0.,0.));
#20091=DIRECTION('center_axis',(0.,-1.,0.));
#20092=DIRECTION('ref_axis',(0.,0.,-1.));
#20093=DIRECTION('center_axis',(6.12323399573676E-17,0.,1.));
#20094=DIRECTION('ref_axis',(1.,0.,0.));
#20095=DIRECTION('center_axis',(0.,-1.,0.));
#20096=DIRECTION('ref_axis',(0.,0.,-1.));
#20097=DIRECTION('center_axis',(0.,1.,0.));
#20098=DIRECTION('ref_axis',(1.,0.,0.));
#20099=DIRECTION('center_axis',(0.,-1.,0.));
#20100=DIRECTION('ref_axis',(1.,0.,0.));
#20101=DIRECTION('center_axis',(0.,-1.,0.));
#20102=DIRECTION('ref_axis',(0.,0.,-1.));
#20103=DIRECTION('center_axis',(0.,0.,1.));
#20104=DIRECTION('ref_axis',(1.,0.,0.));
#20105=DIRECTION('center_axis',(0.,-1.,0.));
#20106=DIRECTION('ref_axis',(0.,0.,-1.));
#20107=DIRECTION('center_axis',(0.,1.,0.));
#20108=DIRECTION('ref_axis',(1.,0.,0.));
#20109=DIRECTION('center_axis',(0.,1.,0.));
#20110=DIRECTION('ref_axis',(1.,0.,0.));
#20111=DIRECTION('',(0.,1.,0.));
#20112=DIRECTION('center_axis',(0.,-1.,0.));
#20113=DIRECTION('ref_axis',(1.,0.,0.));
#20114=DIRECTION('center_axis',(0.,-1.,0.));
#20115=DIRECTION('ref_axis',(1.,0.,0.));
#20116=DIRECTION('center_axis',(0.,1.,0.));
#20117=DIRECTION('ref_axis',(1.,0.,0.));
#20118=DIRECTION('center_axis',(0.,-1.,0.));
#20119=DIRECTION('ref_axis',(0.,0.,-1.));
#20120=DIRECTION('center_axis',(0.,0.,1.));
#20121=DIRECTION('ref_axis',(1.,0.,0.));
#20122=DIRECTION('center_axis',(0.,-1.,0.));
#20123=DIRECTION('ref_axis',(0.,0.,-1.));
#20124=DIRECTION('center_axis',(0.,-1.,0.));
#20125=DIRECTION('ref_axis',(-1.,0.,0.));
#20126=DIRECTION('center_axis',(0.,1.,0.));
#20127=DIRECTION('ref_axis',(1.,0.,0.));
#24609=CARTESIAN_POINT('',(0.,0.,0.));
#24610=CARTESIAN_POINT('Origin',(1.18440385848747,0.,1.18440385848747));
#24611=CARTESIAN_POINT('',(0.846804978391753,-0.07938,1.40825612658882));
#24612=CARTESIAN_POINT('',(1.40825612658882,-0.07938,0.846804978391754));
#24613=CARTESIAN_POINT('Ctrl Pts',(0.846804978391752,-0.0793800000000001,
1.40825612658882));
#24614=CARTESIAN_POINT('Ctrl Pts',(0.854205272175554,-0.123401821157026,
1.40380622184538));
#24615=CARTESIAN_POINT('Ctrl Pts',(0.867957148219441,-0.166543350814306,
1.39550172959303));
#24616=CARTESIAN_POINT('Ctrl Pts',(0.902193646979982,-0.237231147975234,
1.3735491215176));
#24617=CARTESIAN_POINT('Ctrl Pts',(0.920778333482564,-0.266264900654909,
1.36127834356734));
#24618=CARTESIAN_POINT('Ctrl Pts',(0.962485392528369,-0.317195968905306,
1.33211611256184));
#24619=CARTESIAN_POINT('Ctrl Pts',(0.985600426557816,-0.33909093068465,
1.31521005565926));
#24620=CARTESIAN_POINT('Ctrl Pts',(1.03253285680459,-0.373586846396559,
1.27866649102984));
#24621=CARTESIAN_POINT('Ctrl Pts',(1.05871835910697,-0.388086240756494,
1.25722555095714));
#24622=CARTESIAN_POINT('Ctrl Pts',(1.11153475808518,-0.407068917407805,
1.2107812086231));
#24623=CARTESIAN_POINT('Ctrl Pts',(1.13814686046673,-0.411552957311693,
1.18575674747573));
#24624=CARTESIAN_POINT('Ctrl Pts',(1.18575674747573,-0.411552957311693,
1.13814686046673));
#24625=CARTESIAN_POINT('Ctrl Pts',(1.2107812086231,-0.407068917407805,1.11153475808518));
#24626=CARTESIAN_POINT('Ctrl Pts',(1.25722555095713,-0.388086240756494,
1.05871835910697));
#24627=CARTESIAN_POINT('Ctrl Pts',(1.27866649102984,-0.373586846396559,
1.03253285680459));
#24628=CARTESIAN_POINT('Ctrl Pts',(1.31521005565926,-0.33909093068465,0.985600426557816));
#24629=CARTESIAN_POINT('Ctrl Pts',(1.33211611256184,-0.317195968905306,
0.962485392528369));
#24630=CARTESIAN_POINT('Ctrl Pts',(1.36127834356734,-0.266264900654909,
0.920778333482565));
#24631=CARTESIAN_POINT('Ctrl Pts',(1.3735491215176,-0.237231147975234,0.902193646979983));
#24632=CARTESIAN_POINT('Ctrl Pts',(1.39550172959303,-0.166543350814306,
0.867957148219442));
#24633=CARTESIAN_POINT('Ctrl Pts',(1.40380622184538,-0.123401821157026,
0.854205272175555));
#24634=CARTESIAN_POINT('Ctrl Pts',(1.40825612658882,-0.0793800000000001,
0.846804978391753));
#24635=CARTESIAN_POINT('',(0.886256117232623,-0.07938,1.45861320581289));
#24636=CARTESIAN_POINT('Origin',(1.18440385848747,-0.07938,1.18440385848747));
#24637=CARTESIAN_POINT('',(1.45861320581289,-0.07938,0.886256117232624));
#24638=CARTESIAN_POINT('Ctrl Pts',(1.45861320581289,-0.0793800000000001,
0.886256117232623));
#24639=CARTESIAN_POINT('Ctrl Pts',(1.45630208793976,-0.101649918886749,
0.890059788636852));
#24640=CARTESIAN_POINT('Ctrl Pts',(1.45296717977858,-0.123823518623746,
0.895520212222107));
#24641=CARTESIAN_POINT('Ctrl Pts',(1.43904931717599,-0.192480977588836,
0.917859913453975));
#24642=CARTESIAN_POINT('Ctrl Pts',(1.4243271592157,-0.236152929235938,0.940896403863072));
#24643=CARTESIAN_POINT('Ctrl Pts',(1.39055359345152,-0.303141259068212,
0.990027513266106));
#24644=CARTESIAN_POINT('Ctrl Pts',(1.36743459453896,-0.335108247315849,
1.02199477007745));
#24645=CARTESIAN_POINT('Ctrl Pts',(1.32643091652006,-0.373243761060364,
1.07446535104584));
#24646=CARTESIAN_POINT('Ctrl Pts',(1.30441816675528,-0.387888272594439,
1.10126842659597));
#24647=CARTESIAN_POINT('Ctrl Pts',(1.25681160160691,-0.407041111792943,
1.15530234155453));
#24648=CARTESIAN_POINT('Ctrl Pts',(1.23119764287622,-0.411552957311693,
1.18251418313119));
#24649=CARTESIAN_POINT('Ctrl Pts',(1.18251418313119,-0.411552957311693,
1.23119764287622));
#24650=CARTESIAN_POINT('Ctrl Pts',(1.15530234155453,-0.407041111792943,
1.25681160160691));
#24651=CARTESIAN_POINT('Ctrl Pts',(1.10126842659597,-0.387888272594439,
1.30441816675528));
#24652=CARTESIAN_POINT('Ctrl Pts',(1.07446535104584,-0.373243761060364,
1.32643091652006));
#24653=CARTESIAN_POINT('Ctrl Pts',(1.02199477007745,-0.335108247315848,
1.36743459453896));
#24654=CARTESIAN_POINT('Ctrl Pts',(0.990027513266105,-0.303141259068211,
1.39055359345152));
#24655=CARTESIAN_POINT('Ctrl Pts',(0.940896403863071,-0.236152929235937,
1.42432715921571));
#24656=CARTESIAN_POINT('Ctrl Pts',(0.917859913453974,-0.192480977588835,
1.43904931717599));
#24657=CARTESIAN_POINT('Ctrl Pts',(0.895520212222106,-0.123823518623745,
1.45296717977858));
#24658=CARTESIAN_POINT('Ctrl Pts',(0.890059788636851,-0.101649918886749,
1.45630208793976));
#24659=CARTESIAN_POINT('Ctrl Pts',(0.886256117232622,-0.0793800000000001,
1.45861320581289));
#24660=CARTESIAN_POINT('Origin',(1.18440385848747,-0.07938,1.18440385848747));
#24661=CARTESIAN_POINT('Origin',(0.,-0.27783,0.));
#24662=CARTESIAN_POINT('',(0.404717578595295,-0.07938,1.65807299932179));
#24663=CARTESIAN_POINT('Origin',(0.,-0.07938,0.));
#24664=CARTESIAN_POINT('',(-0.404717578595296,-0.07938,1.65807299932179));
#24665=CARTESIAN_POINT('Ctrl Pts',(0.404717578595296,-0.0793800000000001,
1.65807299932179));
#24666=CARTESIAN_POINT('Ctrl Pts',(0.400393769631747,-0.101649918886749,
1.65912839404491));
#24667=CARTESIAN_POINT('Ctrl Pts',(0.394174530911058,-0.123823518623745,
1.66063136041479));
#24668=CARTESIAN_POINT('Ctrl Pts',(0.368536561654407,-0.192480977588835,
1.66658649961961));
#24669=CARTESIAN_POINT('Ctrl Pts',(0.341837165343982,-0.236152929235937,
1.67246562047521));
#24670=CARTESIAN_POINT('Ctrl Pts',(0.283214707341173,-0.303141259068211,
1.68332504372461));
#24671=CARTESIAN_POINT('Ctrl Pts',(0.244262842368623,-0.335108247315849,
1.68958170688653));
#24672=CARTESIAN_POINT('Ctrl Pts',(0.178166559972324,-0.373243761060364,
1.69769003172132));
#24673=CARTESIAN_POINT('Ctrl Pts',(0.143648558862931,-0.387888272594439,
1.70107730356824));
#24674=CARTESIAN_POINT('Ctrl Pts',(0.0717778861362652,-0.407041111792943,
1.70562212620408));
#24675=CARTESIAN_POINT('Ctrl Pts',(0.0344244045173309,-0.411552957311693,
1.706752));
#24676=CARTESIAN_POINT('Ctrl Pts',(-0.0344244045173315,-0.411552957311693,
1.706752));
#24677=CARTESIAN_POINT('Ctrl Pts',(-0.0717778861362658,-0.407041111792943,
1.70562212620408));
#24678=CARTESIAN_POINT('Ctrl Pts',(-0.143648558862932,-0.387888272594439,
1.70107730356824));
#24679=CARTESIAN_POINT('Ctrl Pts',(-0.178166559972325,-0.373243761060364,
1.69769003172132));
#24680=CARTESIAN_POINT('Ctrl Pts',(-0.244262842368624,-0.335108247315849,
1.68958170688653));
#24681=CARTESIAN_POINT('Ctrl Pts',(-0.283214707341173,-0.303141259068212,
1.68332504372461));
#24682=CARTESIAN_POINT('Ctrl Pts',(-0.341837165343982,-0.236152929235937,
1.67246562047521));
#24683=CARTESIAN_POINT('Ctrl Pts',(-0.368536561654408,-0.192480977588835,
1.66658649961961));
#24684=CARTESIAN_POINT('Ctrl Pts',(-0.394174530911059,-0.123823518623745,
1.66063136041479));
#24685=CARTESIAN_POINT('Ctrl Pts',(-0.400393769631748,-0.101649918886749,
1.65912839404491));
#24686=CARTESIAN_POINT('Ctrl Pts',(-0.404717578595297,-0.0793800000000001,
1.65807299932179));
#24687=CARTESIAN_POINT('',(-0.886256117232624,-0.07938,1.45861320581289));
#24688=CARTESIAN_POINT('Origin',(0.,-0.07938,0.));
#24689=CARTESIAN_POINT('',(-1.45861320581289,-0.07938,0.886256117232623));
#24690=CARTESIAN_POINT('Ctrl Pts',(-0.886256117232623,-0.0793800000000001,
1.45861320581289));
#24691=CARTESIAN_POINT('Ctrl Pts',(-0.890059788636852,-0.101649918886749,
1.45630208793976));
#24692=CARTESIAN_POINT('Ctrl Pts',(-0.895520212222106,-0.123823518623745,
1.45296717977858));
#24693=CARTESIAN_POINT('Ctrl Pts',(-0.917859913453974,-0.192480977588835,
1.43904931717599));
#24694=CARTESIAN_POINT('Ctrl Pts',(-0.940896403863071,-0.236152929235937,
1.4243271592157));
#24695=CARTESIAN_POINT('Ctrl Pts',(-0.990027513266105,-0.303141259068211,
1.39055359345152));
#24696=CARTESIAN_POINT('Ctrl Pts',(-1.02199477007745,-0.335108247315848,
1.36743459453896));
#24697=CARTESIAN_POINT('Ctrl Pts',(-1.07446535104584,-0.373243761060364,
1.32643091652006));
#24698=CARTESIAN_POINT('Ctrl Pts',(-1.10126842659597,-0.387888272594439,
1.30441816675528));
#24699=CARTESIAN_POINT('Ctrl Pts',(-1.15530234155453,-0.407041111792943,
1.25681160160691));
#24700=CARTESIAN_POINT('Ctrl Pts',(-1.18251418313119,-0.411552957311693,
1.23119764287622));
#24701=CARTESIAN_POINT('Ctrl Pts',(-1.23119764287622,-0.411552957311693,
1.18251418313119));
#24702=CARTESIAN_POINT('Ctrl Pts',(-1.25681160160691,-0.407041111792943,
1.15530234155453));
#24703=CARTESIAN_POINT('Ctrl Pts',(-1.30441816675528,-0.387888272594439,
1.10126842659597));
#24704=CARTESIAN_POINT('Ctrl Pts',(-1.32643091652006,-0.373243761060365,
1.07446535104584));
#24705=CARTESIAN_POINT('Ctrl Pts',(-1.36743459453896,-0.335108247315849,
1.02199477007745));
#24706=CARTESIAN_POINT('Ctrl Pts',(-1.39055359345152,-0.303141259068212,
0.990027513266106));
#24707=CARTESIAN_POINT('Ctrl Pts',(-1.4243271592157,-0.236152929235938,
0.940896403863071));
#24708=CARTESIAN_POINT('Ctrl Pts',(-1.43904931717599,-0.192480977588836,
0.917859913453974));
#24709=CARTESIAN_POINT('Ctrl Pts',(-1.45296717977858,-0.123823518623746,
0.895520212222106));
#24710=CARTESIAN_POINT('Ctrl Pts',(-1.45630208793976,-0.101649918886749,
0.890059788636852));
#24711=CARTESIAN_POINT('Ctrl Pts',(-1.45861320581289,-0.0793800000000001,
0.886256117232623));
#24712=CARTESIAN_POINT('',(-1.65807299932179,-0.07938,0.404717578595295));
#24713=CARTESIAN_POINT('Origin',(0.,-0.07938,0.));
#24714=CARTESIAN_POINT('',(-1.706752,-0.411552957311693,2.08591827245526E-16));
#24715=CARTESIAN_POINT('Ctrl Pts',(-1.65807299932179,-0.0793800000000001,
0.404717578595296));
#24716=CARTESIAN_POINT('Ctrl Pts',(-1.65912839404491,-0.101649918886749,
0.400393769631747));
#24717=CARTESIAN_POINT('Ctrl Pts',(-1.66063136041479,-0.123823518623745,
0.394174530911058));
#24718=CARTESIAN_POINT('Ctrl Pts',(-1.66658649961961,-0.192480977588835,
0.368536561654407));
#24719=CARTESIAN_POINT('Ctrl Pts',(-1.67246562047521,-0.236152929235937,
0.341837165343982));
#24720=CARTESIAN_POINT('Ctrl Pts',(-1.68332504372461,-0.303141259068211,
0.283214707341173));
#24721=CARTESIAN_POINT('Ctrl Pts',(-1.68958170688653,-0.335108247315848,
0.244262842368623));
#24722=CARTESIAN_POINT('Ctrl Pts',(-1.69769003172132,-0.373243761060364,
0.178166559972324));
#24723=CARTESIAN_POINT('Ctrl Pts',(-1.70107730356824,-0.387888272594439,
0.143648558862931));
#24724=CARTESIAN_POINT('Ctrl Pts',(-1.70562212620408,-0.407041111792943,
0.0717778861362656));
#24725=CARTESIAN_POINT('Ctrl Pts',(-1.706752,-0.411552957311693,0.0344244045173313));
#24726=CARTESIAN_POINT('Ctrl Pts',(-1.706752,-0.411552957311693,2.08166817117217E-16));
#24727=CARTESIAN_POINT('',(-1.706752,-0.47628,2.09016837373834E-16));
#24728=CARTESIAN_POINT('',(-1.706752,-0.27783,2.09016837373834E-16));
#24729=CARTESIAN_POINT('Origin',(0.,-0.47628,0.));
#24730=CARTESIAN_POINT('',(-1.65807299932179,-0.07938,-0.404717578595296));
#24731=CARTESIAN_POINT('Ctrl Pts',(-1.706752,-0.411552957311693,2.0122792321331E-16));
#24732=CARTESIAN_POINT('Ctrl Pts',(-1.706752,-0.411552957311693,-0.0344244045173309));
#24733=CARTESIAN_POINT('Ctrl Pts',(-1.70562212620408,-0.407041111792943,
-0.0717778861362652));
#24734=CARTESIAN_POINT('Ctrl Pts',(-1.70107730356824,-0.387888272594439,
-0.143648558862931));
#24735=CARTESIAN_POINT('Ctrl Pts',(-1.69769003172132,-0.373243761060365,
-0.178166559972324));
#24736=CARTESIAN_POINT('Ctrl Pts',(-1.68958170688653,-0.335108247315849,
-0.244262842368623));
#24737=CARTESIAN_POINT('Ctrl Pts',(-1.68332504372461,-0.303141259068212,
-0.283214707341173));
#24738=CARTESIAN_POINT('Ctrl Pts',(-1.67246562047521,-0.236152929235938,
-0.341837165343982));
#24739=CARTESIAN_POINT('Ctrl Pts',(-1.66658649961961,-0.192480977588836,
-0.368536561654407));
#24740=CARTESIAN_POINT('Ctrl Pts',(-1.66063136041479,-0.123823518623745,
-0.394174530911059));
#24741=CARTESIAN_POINT('Ctrl Pts',(-1.65912839404491,-0.101649918886749,
-0.400393769631748));
#24742=CARTESIAN_POINT('Ctrl Pts',(-1.65807299932179,-0.0793800000000001,
-0.404717578595296));
#24743=CARTESIAN_POINT('',(-1.45861320581289,-0.07938,-0.886256117232623));
#24744=CARTESIAN_POINT('Origin',(0.,-0.07938,0.));
#24745=CARTESIAN_POINT('',(-0.886256117232623,-0.07938,-1.45861320581289));
#24746=CARTESIAN_POINT('Ctrl Pts',(-1.45861320581289,-0.0793800000000001,
-0.886256117232623));
#24747=CARTESIAN_POINT('Ctrl Pts',(-1.45630208793976,-0.101649918886749,
-0.890059788636852));
#24748=CARTESIAN_POINT('Ctrl Pts',(-1.45296717977858,-0.123823518623745,
-0.895520212222106));
#24749=CARTESIAN_POINT('Ctrl Pts',(-1.43904931717599,-0.192480977588835,
-0.917859913453974));
#24750=CARTESIAN_POINT('Ctrl Pts',(-1.4243271592157,-0.236152929235937,
-0.940896403863072));
#24751=CARTESIAN_POINT('Ctrl Pts',(-1.39055359345152,-0.303141259068212,
-0.990027513266106));
#24752=CARTESIAN_POINT('Ctrl Pts',(-1.36743459453896,-0.335108247315849,
-1.02199477007745));
#24753=CARTESIAN_POINT('Ctrl Pts',(-1.32643091652006,-0.373243761060364,
-1.07446535104584));
#24754=CARTESIAN_POINT('Ctrl Pts',(-1.30441816675528,-0.387888272594439,
-1.10126842659597));
#24755=CARTESIAN_POINT('Ctrl Pts',(-1.25681160160691,-0.407041111792943,
-1.15530234155453));
#24756=CARTESIAN_POINT('Ctrl Pts',(-1.23119764287622,-0.411552957311693,
-1.18251418313119));
#24757=CARTESIAN_POINT('Ctrl Pts',(-1.18251418313119,-0.411552957311693,
-1.23119764287622));
#24758=CARTESIAN_POINT('Ctrl Pts',(-1.15530234155453,-0.407041111792943,
-1.25681160160691));
#24759=CARTESIAN_POINT('Ctrl Pts',(-1.10126842659597,-0.387888272594439,
-1.30441816675528));
#24760=CARTESIAN_POINT('Ctrl Pts',(-1.07446535104584,-0.373243761060364,
-1.32643091652006));
#24761=CARTESIAN_POINT('Ctrl Pts',(-1.02199477007745,-0.335108247315848,
-1.36743459453896));
#24762=CARTESIAN_POINT('Ctrl Pts',(-0.990027513266105,-0.303141259068211,
-1.39055359345152));
#24763=CARTESIAN_POINT('Ctrl Pts',(-0.940896403863071,-0.236152929235936,
-1.42432715921571));
#24764=CARTESIAN_POINT('Ctrl Pts',(-0.917859913453974,-0.192480977588835,
-1.43904931717599));
#24765=CARTESIAN_POINT('Ctrl Pts',(-0.895520212222106,-0.123823518623745,
-1.45296717977858));
#24766=CARTESIAN_POINT('Ctrl Pts',(-0.890059788636851,-0.101649918886749,
-1.45630208793976));
#24767=CARTESIAN_POINT('Ctrl Pts',(-0.886256117232623,-0.0793800000000001,
-1.45861320581289));
#24768=CARTESIAN_POINT('',(-0.404717578595295,-0.07938,-1.65807299932179));
#24769=CARTESIAN_POINT('Origin',(0.,-0.07938,0.));
#24770=CARTESIAN_POINT('',(0.404717578595296,-0.07938,-1.65807299932179));
#24771=CARTESIAN_POINT('Ctrl Pts',(-0.404717578595296,-0.0793800000000001,
-1.65807299932179));
#24772=CARTESIAN_POINT('Ctrl Pts',(-0.400393769631747,-0.101649918886749,
-1.65912839404491));
#24773=CARTESIAN_POINT('Ctrl Pts',(-0.394174530911058,-0.123823518623746,
-1.66063136041479));
#24774=CARTESIAN_POINT('Ctrl Pts',(-0.368536561654407,-0.192480977588836,
-1.66658649961961));
#24775=CARTESIAN_POINT('Ctrl Pts',(-0.341837165343982,-0.236152929235938,
-1.67246562047521));
#24776=CARTESIAN_POINT('Ctrl Pts',(-0.283214707341173,-0.303141259068212,
-1.68332504372461));
#24777=CARTESIAN_POINT('Ctrl Pts',(-0.244262842368623,-0.335108247315849,
-1.68958170688653));
#24778=CARTESIAN_POINT('Ctrl Pts',(-0.178166559972324,-0.373243761060364,
-1.69769003172132));
#24779=CARTESIAN_POINT('Ctrl Pts',(-0.143648558862931,-0.387888272594439,
-1.70107730356824));
#24780=CARTESIAN_POINT('Ctrl Pts',(-0.0717778861362653,-0.407041111792943,
-1.70562212620408));
#24781=CARTESIAN_POINT('Ctrl Pts',(-0.034424404517331,-0.411552957311693,
-1.706752));
#24782=CARTESIAN_POINT('Ctrl Pts',(0.0344244045173312,-0.411552957311693,
-1.706752));
#24783=CARTESIAN_POINT('Ctrl Pts',(0.0717778861362655,-0.407041111792943,
-1.70562212620408));
#24784=CARTESIAN_POINT('Ctrl Pts',(0.143648558862931,-0.387888272594439,
-1.70107730356824));
#24785=CARTESIAN_POINT('Ctrl Pts',(0.178166559972324,-0.373243761060364,
-1.69769003172132));
#24786=CARTESIAN_POINT('Ctrl Pts',(0.244262842368623,-0.335108247315849,
-1.68958170688653));
#24787=CARTESIAN_POINT('Ctrl Pts',(0.283214707341173,-0.303141259068212,
-1.68332504372461));
#24788=CARTESIAN_POINT('Ctrl Pts',(0.341837165343982,-0.236152929235937,
-1.67246562047521));
#24789=CARTESIAN_POINT('Ctrl Pts',(0.368536561654407,-0.192480977588835,
-1.66658649961961));
#24790=CARTESIAN_POINT('Ctrl Pts',(0.394174530911059,-0.123823518623745,
-1.66063136041479));
#24791=CARTESIAN_POINT('Ctrl Pts',(0.400393769631748,-0.101649918886749,
-1.65912839404491));
#24792=CARTESIAN_POINT('Ctrl Pts',(0.404717578595296,-0.0793800000000001,
-1.65807299932179));
#24793=CARTESIAN_POINT('',(0.886256117232623,-0.07938,-1.45861320581289));
#24794=CARTESIAN_POINT('Origin',(0.,-0.07938,0.));
#24795=CARTESIAN_POINT('',(1.45861320581289,-0.07938,-0.886256117232623));
#24796=CARTESIAN_POINT('Ctrl Pts',(0.886256117232623,-0.0793800000000001,
-1.45861320581289));
#24797=CARTESIAN_POINT('Ctrl Pts',(0.890059788636852,-0.101649918886749,
-1.45630208793976));
#24798=CARTESIAN_POINT('Ctrl Pts',(0.895520212222106,-0.123823518623745,
-1.45296717977858));
#24799=CARTESIAN_POINT('Ctrl Pts',(0.917859913453974,-0.192480977588835,
-1.43904931717599));
#24800=CARTESIAN_POINT('Ctrl Pts',(0.940896403863072,-0.236152929235937,
-1.4243271592157));
#24801=CARTESIAN_POINT('Ctrl Pts',(0.990027513266106,-0.303141259068211,
-1.39055359345152));
#24802=CARTESIAN_POINT('Ctrl Pts',(1.02199477007745,-0.335108247315849,
-1.36743459453896));
#24803=CARTESIAN_POINT('Ctrl Pts',(1.07446535104584,-0.373243761060364,
-1.32643091652006));
#24804=CARTESIAN_POINT('Ctrl Pts',(1.10126842659597,-0.387888272594439,
-1.30441816675528));
#24805=CARTESIAN_POINT('Ctrl Pts',(1.15530234155453,-0.407041111792943,
-1.25681160160691));
#24806=CARTESIAN_POINT('Ctrl Pts',(1.18251418313119,-0.411552957311693,
-1.23119764287622));
#24807=CARTESIAN_POINT('Ctrl Pts',(1.23119764287622,-0.411552957311693,
-1.18251418313119));
#24808=CARTESIAN_POINT('Ctrl Pts',(1.25681160160691,-0.407041111792943,
-1.15530234155453));
#24809=CARTESIAN_POINT('Ctrl Pts',(1.30441816675528,-0.387888272594439,
-1.10126842659597));
#24810=CARTESIAN_POINT('Ctrl Pts',(1.32643091652006,-0.373243761060364,
-1.07446535104584));
#24811=CARTESIAN_POINT('Ctrl Pts',(1.36743459453896,-0.335108247315849,
-1.02199477007745));
#24812=CARTESIAN_POINT('Ctrl Pts',(1.39055359345152,-0.303141259068212,
-0.990027513266105));
#24813=CARTESIAN_POINT('Ctrl Pts',(1.4243271592157,-0.236152929235937,-0.940896403863071));
#24814=CARTESIAN_POINT('Ctrl Pts',(1.43904931717599,-0.192480977588835,
-0.917859913453974));
#24815=CARTESIAN_POINT('Ctrl Pts',(1.45296717977858,-0.123823518623745,
-0.895520212222106));
#24816=CARTESIAN_POINT('Ctrl Pts',(1.45630208793976,-0.101649918886749,
-0.890059788636852));
#24817=CARTESIAN_POINT('Ctrl Pts',(1.45861320581289,-0.0793800000000001,
-0.886256117232623));
#24818=CARTESIAN_POINT('',(1.65807299932179,-0.07938,-0.404717578595296));
#24819=CARTESIAN_POINT('Origin',(0.,-0.07938,0.));
#24820=CARTESIAN_POINT('',(1.65807299932179,-0.07938,0.404717578595296));
#24821=CARTESIAN_POINT('Ctrl Pts',(1.65807299932179,-0.0793800000000001,
-0.404717578595296));
#24822=CARTESIAN_POINT('Ctrl Pts',(1.65912839404491,-0.101649918886749,
-0.400393769631747));
#24823=CARTESIAN_POINT('Ctrl Pts',(1.66063136041479,-0.123823518623745,
-0.394174530911058));
#24824=CARTESIAN_POINT('Ctrl Pts',(1.66658649961961,-0.192480977588835,
-0.368536561654407));
#24825=CARTESIAN_POINT('Ctrl Pts',(1.67246562047521,-0.236152929235937,
-0.341837165343982));
#24826=CARTESIAN_POINT('Ctrl Pts',(1.68332504372461,-0.303141259068212,
-0.283214707341173));
#24827=CARTESIAN_POINT('Ctrl Pts',(1.68958170688653,-0.335108247315849,
-0.244262842368623));
#24828=CARTESIAN_POINT('Ctrl Pts',(1.69769003172132,-0.373243761060364,
-0.178166559972324));
#24829=CARTESIAN_POINT('Ctrl Pts',(1.70107730356824,-0.387888272594439,
-0.143648558862931));
#24830=CARTESIAN_POINT('Ctrl Pts',(1.70562212620408,-0.407041111792943,
-0.0717778861362655));
#24831=CARTESIAN_POINT('Ctrl Pts',(1.706752,-0.411552957311693,-0.0344244045173312));
#24832=CARTESIAN_POINT('Ctrl Pts',(1.706752,-0.411552957311693,0.0344244045173312));
#24833=CARTESIAN_POINT('Ctrl Pts',(1.70562212620408,-0.407041111792943,
0.0717778861362655));
#24834=CARTESIAN_POINT('Ctrl Pts',(1.70107730356824,-0.387888272594439,
0.143648558862931));
#24835=CARTESIAN_POINT('Ctrl Pts',(1.69769003172132,-0.373243761060364,
0.178166559972324));
#24836=CARTESIAN_POINT('Ctrl Pts',(1.68958170688653,-0.335108247315849,
0.244262842368623));
#24837=CARTESIAN_POINT('Ctrl Pts',(1.68332504372461,-0.303141259068212,
0.283214707341173));
#24838=CARTESIAN_POINT('Ctrl Pts',(1.67246562047521,-0.236152929235937,
0.341837165343982));
#24839=CARTESIAN_POINT('Ctrl Pts',(1.66658649961961,-0.192480977588835,
0.368536561654407));
#24840=CARTESIAN_POINT('Ctrl Pts',(1.66063136041479,-0.123823518623745,
0.394174530911058));
#24841=CARTESIAN_POINT('Ctrl Pts',(1.65912839404491,-0.101649918886749,
0.400393769631747));
#24842=CARTESIAN_POINT('Ctrl Pts',(1.65807299932179,-0.0793800000000001,
0.404717578595296));
#24843=CARTESIAN_POINT('Origin',(0.,-0.07938,0.));
#24844=CARTESIAN_POINT('Origin',(0.,-0.07938,0.));
#24845=CARTESIAN_POINT('',(0.397005914195118,-0.07938,1.59456899932179));
#24846=CARTESIAN_POINT('Origin',(0.,-0.07938,0.));
#24847=CARTESIAN_POINT('Origin',(-3.33066907387547E-16,-0.07938,1.675));
#24848=CARTESIAN_POINT('Origin',(-3.33066907387547E-16,0.,1.675));
#24849=CARTESIAN_POINT('',(-0.397005914195118,-0.07938,1.59456899932179));
#24850=CARTESIAN_POINT('Ctrl Pts',(-0.397005914195119,-0.0793800000000001,
1.59456899932179));
#24851=CARTESIAN_POINT('Ctrl Pts',(-0.3886265584581,-0.123401821157026,
1.59665523941937));
#24852=CARTESIAN_POINT('Ctrl Pts',(-0.373030350867485,-0.166543350814306,
1.60050712143809));
#24853=CARTESIAN_POINT('Ctrl Pts',(-0.333298652394954,-0.237231147975234,
1.60919314384089));
#24854=CARTESIAN_POINT('Ctrl Pts',(-0.311480544243687,-0.266264900654909,
1.61365775139403));
#24855=CARTESIAN_POINT('Ctrl Pts',(-0.261368388670537,-0.317195968905306,
1.62252828437015));
#24856=CARTESIAN_POINT('Ctrl Pts',(-0.233069203882014,-0.33909093068465,
1.62691869420078));
#24857=CARTESIAN_POINT('Ctrl Pts',(-0.174042761838764,-0.373586846396559,
1.63426473152765));
#24858=CARTESIAN_POINT('Ctrl Pts',(-0.14036578147155,-0.388086240756494,
1.63761964365402));
#24859=CARTESIAN_POINT('Ctrl Pts',(-0.0701778381840615,-0.407068917407805,
1.64212536811722));
#24860=CARTESIAN_POINT('Ctrl Pts',(-0.0336652739555918,-0.411552957311693,
1.643248));
#24861=CARTESIAN_POINT('Ctrl Pts',(0.0336652739555913,-0.411552957311693,
1.643248));
#24862=CARTESIAN_POINT('Ctrl Pts',(0.070177838184061,-0.407068917407805,
1.64212536811722));
#24863=CARTESIAN_POINT('Ctrl Pts',(0.140365781471549,-0.388086240756494,
1.63761964365402));
#24864=CARTESIAN_POINT('Ctrl Pts',(0.174042761838763,-0.373586846396559,
1.63426473152765));
#24865=CARTESIAN_POINT('Ctrl Pts',(0.233069203882014,-0.33909093068465,
1.62691869420078));
#24866=CARTESIAN_POINT('Ctrl Pts',(0.261368388670536,-0.317195968905306,
1.62252828437015));
#24867=CARTESIAN_POINT('Ctrl Pts',(0.311480544243686,-0.266264900654908,
1.61365775139403));
#24868=CARTESIAN_POINT('Ctrl Pts',(0.333298652394954,-0.237231147975234,
1.60919314384089));
#24869=CARTESIAN_POINT('Ctrl Pts',(0.373030350867484,-0.166543350814306,
1.60050712143809));
#24870=CARTESIAN_POINT('Ctrl Pts',(0.388626558458099,-0.123401821157026,
1.59665523941937));
#24871=CARTESIAN_POINT('Ctrl Pts',(0.397005914195118,-0.07938,1.59456899932179));
#24872=CARTESIAN_POINT('Origin',(-3.33066907387547E-16,-0.07938,1.675));
#24873=CARTESIAN_POINT('Origin',(0.,-0.07938,0.));
#24874=CARTESIAN_POINT('',(-0.846804978391754,-0.07938,1.40825612658882));
#24875=CARTESIAN_POINT('Origin',(0.,-0.07938,0.));
#24876=CARTESIAN_POINT('Origin',(-1.18440385848747,-0.07938,1.18440385848747));
#24877=CARTESIAN_POINT('Origin',(-1.18440385848747,0.,1.18440385848747));
#24878=CARTESIAN_POINT('',(-1.40825612658882,-0.07938,0.846804978391753));
#24879=CARTESIAN_POINT('Ctrl Pts',(-1.40825612658882,-0.0793800000000001,
0.846804978391753));
#24880=CARTESIAN_POINT('Ctrl Pts',(-1.40380622184538,-0.123401821157026,
0.854205272175555));
#24881=CARTESIAN_POINT('Ctrl Pts',(-1.39550172959303,-0.166543350814306,
0.867957148219442));
#24882=CARTESIAN_POINT('Ctrl Pts',(-1.3735491215176,-0.237231147975235,
0.902193646979983));
#24883=CARTESIAN_POINT('Ctrl Pts',(-1.36127834356734,-0.266264900654909,
0.920778333482565));
#24884=CARTESIAN_POINT('Ctrl Pts',(-1.33211611256184,-0.317195968905306,
0.962485392528369));
#24885=CARTESIAN_POINT('Ctrl Pts',(-1.31521005565926,-0.339090930684651,
0.985600426557816));
#24886=CARTESIAN_POINT('Ctrl Pts',(-1.27866649102984,-0.373586846396559,
1.03253285680459));
#24887=CARTESIAN_POINT('Ctrl Pts',(-1.25722555095714,-0.388086240756494,
1.05871835910697));
#24888=CARTESIAN_POINT('Ctrl Pts',(-1.2107812086231,-0.407068917407805,
1.11153475808518));
#24889=CARTESIAN_POINT('Ctrl Pts',(-1.18575674747573,-0.411552957311693,
1.13814686046673));
#24890=CARTESIAN_POINT('Ctrl Pts',(-1.13814686046673,-0.411552957311693,
1.18575674747573));
#24891=CARTESIAN_POINT('Ctrl Pts',(-1.11153475808518,-0.407068917407805,
1.2107812086231));
#24892=CARTESIAN_POINT('Ctrl Pts',(-1.05871835910697,-0.388086240756494,
1.25722555095714));
#24893=CARTESIAN_POINT('Ctrl Pts',(-1.03253285680459,-0.373586846396559,
1.27866649102984));
#24894=CARTESIAN_POINT('Ctrl Pts',(-0.985600426557816,-0.33909093068465,
1.31521005565926));
#24895=CARTESIAN_POINT('Ctrl Pts',(-0.962485392528369,-0.317195968905306,
1.33211611256184));
#24896=CARTESIAN_POINT('Ctrl Pts',(-0.920778333482565,-0.266264900654908,
1.36127834356734));
#24897=CARTESIAN_POINT('Ctrl Pts',(-0.902193646979983,-0.237231147975234,
1.3735491215176));
#24898=CARTESIAN_POINT('Ctrl Pts',(-0.867957148219442,-0.166543350814306,
1.39550172959303));
#24899=CARTESIAN_POINT('Ctrl Pts',(-0.854205272175555,-0.123401821157026,
1.40380622184538));
#24900=CARTESIAN_POINT('Ctrl Pts',(-0.846804978391753,-0.0793800000000001,
1.40825612658882));
#24901=CARTESIAN_POINT('Origin',(-1.18440385848747,-0.07938,1.18440385848747));
#24902=CARTESIAN_POINT('Origin',(0.,-0.07938,0.));
#24903=CARTESIAN_POINT('',(-1.59456899932179,-0.07938,0.397005914195118));
#24904=CARTESIAN_POINT('Origin',(0.,-0.07938,0.));
#24905=CARTESIAN_POINT('Origin',(-1.675,-0.07938,-2.22044604925031E-16));
#24906=CARTESIAN_POINT('Origin',(-1.675,0.,-2.22044604925031E-16));
#24907=CARTESIAN_POINT('',(-1.59456899932179,-0.07938,-0.397005914195118));
#24908=CARTESIAN_POINT('',(-1.643248,-0.411552957311693,3.47540551556327E-18));
#24909=CARTESIAN_POINT('Ctrl Pts',(-1.59456899932179,-0.0793800000000001,
-0.397005914195119));
#24910=CARTESIAN_POINT('Ctrl Pts',(-1.59665523941937,-0.123401821157026,
-0.388626558458099));
#24911=CARTESIAN_POINT('Ctrl Pts',(-1.60050712143809,-0.166543350814306,
-0.373030350867485));
#24912=CARTESIAN_POINT('Ctrl Pts',(-1.60919314384089,-0.237231147975234,
-0.333298652394954));
#24913=CARTESIAN_POINT('Ctrl Pts',(-1.61365775139403,-0.266264900654909,
-0.311480544243686));
#24914=CARTESIAN_POINT('Ctrl Pts',(-1.62252828437015,-0.317195968905306,
-0.261368388670537));
#24915=CARTESIAN_POINT('Ctrl Pts',(-1.62691869420078,-0.33909093068465,
-0.233069203882014));
#24916=CARTESIAN_POINT('Ctrl Pts',(-1.63426473152765,-0.373586846396559,
-0.174042761838764));
#24917=CARTESIAN_POINT('Ctrl Pts',(-1.63761964365402,-0.388086240756494,
-0.140365781471549));
#24918=CARTESIAN_POINT('Ctrl Pts',(-1.64212536811722,-0.407068917407805,
-0.0701778381840614));
#24919=CARTESIAN_POINT('Ctrl Pts',(-1.643248,-0.411552957311693,-0.0336652739555917));
#24920=CARTESIAN_POINT('Ctrl Pts',(-1.643248,-0.411552957311693,-2.0122792321331E-16));
#24921=CARTESIAN_POINT('Origin',(-1.675,-0.07938,-2.22044604925031E-16));
#24922=CARTESIAN_POINT('Ctrl Pts',(-1.643248,-0.411552957311693,-1.94289029309402E-16));
#24923=CARTESIAN_POINT('Ctrl Pts',(-1.643248,-0.411552957311693,0.0336652739555913));
#24924=CARTESIAN_POINT('Ctrl Pts',(-1.64212536811722,-0.407068917407805,
0.0701778381840609));
#24925=CARTESIAN_POINT('Ctrl Pts',(-1.63761964365402,-0.388086240756494,
0.140365781471549));
#24926=CARTESIAN_POINT('Ctrl Pts',(-1.63426473152765,-0.373586846396559,
0.174042761838763));
#24927=CARTESIAN_POINT('Ctrl Pts',(-1.62691869420078,-0.33909093068465,
0.233069203882014));
#24928=CARTESIAN_POINT('Ctrl Pts',(-1.62252828437015,-0.317195968905306,
0.261368388670536));
#24929=CARTESIAN_POINT('Ctrl Pts',(-1.61365775139403,-0.266264900654909,
0.311480544243686));
#24930=CARTESIAN_POINT('Ctrl Pts',(-1.60919314384089,-0.237231147975235,
0.333298652394954));
#24931=CARTESIAN_POINT('Ctrl Pts',(-1.60050712143809,-0.166543350814306,
0.373030350867484));
#24932=CARTESIAN_POINT('Ctrl Pts',(-1.59665523941937,-0.123401821157026,
0.388626558458099));
#24933=CARTESIAN_POINT('Ctrl Pts',(-1.59456899932179,-0.0793800000000001,
0.397005914195118));
#24934=CARTESIAN_POINT('Origin',(0.,-0.07938,0.));
#24935=CARTESIAN_POINT('',(-1.40825612658882,-0.07938,-0.846804978391753));
#24936=CARTESIAN_POINT('Origin',(0.,-0.07938,0.));
#24937=CARTESIAN_POINT('Origin',(-1.18440385848747,-0.07938,-1.18440385848747));
#24938=CARTESIAN_POINT('Origin',(-1.18440385848747,0.,-1.18440385848747));
#24939=CARTESIAN_POINT('',(-0.846804978391753,-0.07938,-1.40825612658882));
#24940=CARTESIAN_POINT('Ctrl Pts',(-0.846804978391753,-0.0793800000000001,
-1.40825612658882));
#24941=CARTESIAN_POINT('Ctrl Pts',(-0.854205272175555,-0.123401821157026,
-1.40380622184538));
#24942=CARTESIAN_POINT('Ctrl Pts',(-0.867957148219442,-0.166543350814306,
-1.39550172959303));
#24943=CARTESIAN_POINT('Ctrl Pts',(-0.902193646979982,-0.237231147975234,
-1.3735491215176));
#24944=CARTESIAN_POINT('Ctrl Pts',(-0.920778333482564,-0.266264900654908,
-1.36127834356734));
#24945=CARTESIAN_POINT('Ctrl Pts',(-0.962485392528368,-0.317195968905306,
-1.33211611256184));
#24946=CARTESIAN_POINT('Ctrl Pts',(-0.985600426557816,-0.33909093068465,
-1.31521005565926));
#24947=CARTESIAN_POINT('Ctrl Pts',(-1.03253285680459,-0.373586846396559,
-1.27866649102984));
#24948=CARTESIAN_POINT('Ctrl Pts',(-1.05871835910697,-0.388086240756494,
-1.25722555095714));
#24949=CARTESIAN_POINT('Ctrl Pts',(-1.11153475808518,-0.407068917407805,
-1.2107812086231));
#24950=CARTESIAN_POINT('Ctrl Pts',(-1.13814686046673,-0.411552957311693,
-1.18575674747573));
#24951=CARTESIAN_POINT('Ctrl Pts',(-1.18575674747573,-0.411552957311693,
-1.13814686046673));
#24952=CARTESIAN_POINT('Ctrl Pts',(-1.2107812086231,-0.407068917407805,
-1.11153475808518));
#24953=CARTESIAN_POINT('Ctrl Pts',(-1.25722555095714,-0.388086240756494,
-1.05871835910697));
#24954=CARTESIAN_POINT('Ctrl Pts',(-1.27866649102984,-0.373586846396559,
-1.03253285680459));
#24955=CARTESIAN_POINT('Ctrl Pts',(-1.31521005565926,-0.33909093068465,
-0.985600426557816));
#24956=CARTESIAN_POINT('Ctrl Pts',(-1.33211611256184,-0.317195968905306,
-0.962485392528369));
#24957=CARTESIAN_POINT('Ctrl Pts',(-1.36127834356734,-0.266264900654909,
-0.920778333482565));
#24958=CARTESIAN_POINT('Ctrl Pts',(-1.3735491215176,-0.237231147975234,
-0.902193646979983));
#24959=CARTESIAN_POINT('Ctrl Pts',(-1.39550172959303,-0.166543350814306,
-0.867957148219442));
#24960=CARTESIAN_POINT('Ctrl Pts',(-1.40380622184538,-0.123401821157026,
-0.854205272175555));
#24961=CARTESIAN_POINT('Ctrl Pts',(-1.40825612658882,-0.07938,-0.846804978391753));
#24962=CARTESIAN_POINT('Origin',(-1.18440385848747,-0.07938,-1.18440385848747));
#24963=CARTESIAN_POINT('Origin',(0.,-0.07938,0.));
#24964=CARTESIAN_POINT('',(-0.397005914195118,-0.07938,-1.59456899932179));
#24965=CARTESIAN_POINT('Origin',(0.,-0.07938,0.));
#24966=CARTESIAN_POINT('Origin',(1.11022302462516E-16,-0.07938,-1.675));
#24967=CARTESIAN_POINT('Origin',(1.11022302462516E-16,0.,-1.675));
#24968=CARTESIAN_POINT('',(0.397005914195118,-0.07938,-1.59456899932179));
#24969=CARTESIAN_POINT('Ctrl Pts',(0.397005914195119,-0.0793800000000001,
-1.59456899932179));
#24970=CARTESIAN_POINT('Ctrl Pts',(0.388626558458099,-0.123401821157026,
-1.59665523941937));
#24971=CARTESIAN_POINT('Ctrl Pts',(0.373030350867485,-0.166543350814306,
-1.60050712143809));
#24972=CARTESIAN_POINT('Ctrl Pts',(0.333298652394954,-0.237231147975234,
-1.60919314384089));
#24973=CARTESIAN_POINT('Ctrl Pts',(0.311480544243686,-0.266264900654909,
-1.61365775139403));
#24974=CARTESIAN_POINT('Ctrl Pts',(0.261368388670537,-0.317195968905306,
-1.62252828437015));
#24975=CARTESIAN_POINT('Ctrl Pts',(0.233069203882014,-0.33909093068465,
-1.62691869420078));
#24976=CARTESIAN_POINT('Ctrl Pts',(0.174042761838763,-0.373586846396559,
-1.63426473152765));
#24977=CARTESIAN_POINT('Ctrl Pts',(0.140365781471549,-0.388086240756494,
-1.63761964365402));
#24978=CARTESIAN_POINT('Ctrl Pts',(0.0701778381840612,-0.407068917407805,
-1.64212536811722));
#24979=CARTESIAN_POINT('Ctrl Pts',(0.0336652739555916,-0.411552957311693,
-1.643248));
#24980=CARTESIAN_POINT('Ctrl Pts',(-0.0336652739555915,-0.411552957311693,
-1.643248));
#24981=CARTESIAN_POINT('Ctrl Pts',(-0.0701778381840612,-0.407068917407805,
-1.64212536811722));
#24982=CARTESIAN_POINT('Ctrl Pts',(-0.140365781471549,-0.388086240756494,
-1.63761964365402));
#24983=CARTESIAN_POINT('Ctrl Pts',(-0.174042761838764,-0.373586846396559,
-1.63426473152765));
#24984=CARTESIAN_POINT('Ctrl Pts',(-0.233069203882014,-0.33909093068465,
-1.62691869420078));
#24985=CARTESIAN_POINT('Ctrl Pts',(-0.261368388670536,-0.317195968905306,
-1.62252828437015));
#24986=CARTESIAN_POINT('Ctrl Pts',(-0.311480544243686,-0.266264900654908,
-1.61365775139403));
#24987=CARTESIAN_POINT('Ctrl Pts',(-0.333298652394954,-0.237231147975234,
-1.60919314384089));
#24988=CARTESIAN_POINT('Ctrl Pts',(-0.373030350867485,-0.166543350814306,
-1.60050712143809));
#24989=CARTESIAN_POINT('Ctrl Pts',(-0.388626558458099,-0.123401821157026,
-1.59665523941937));
#24990=CARTESIAN_POINT('Ctrl Pts',(-0.397005914195118,-0.07938,-1.59456899932179));
#24991=CARTESIAN_POINT('Origin',(1.11022302462516E-16,-0.07938,-1.675));
#24992=CARTESIAN_POINT('Origin',(0.,-0.07938,0.));
#24993=CARTESIAN_POINT('',(0.846804978391753,-0.07938,-1.40825612658882));
#24994=CARTESIAN_POINT('Origin',(0.,-0.07938,0.));
#24995=CARTESIAN_POINT('Origin',(1.18440385848747,-0.07938,-1.18440385848747));
#24996=CARTESIAN_POINT('Origin',(1.18440385848747,0.,-1.18440385848747));
#24997=CARTESIAN_POINT('',(1.40825612658882,-0.07938,-0.846804978391753));
#24998=CARTESIAN_POINT('Ctrl Pts',(1.40825612658882,-0.0793800000000001,
-0.846804978391753));
#24999=CARTESIAN_POINT('Ctrl Pts',(1.40380622184538,-0.123401821157026,
-0.854205272175555));
#25000=CARTESIAN_POINT('Ctrl Pts',(1.39550172959303,-0.166543350814306,
-0.867957148219442));
#25001=CARTESIAN_POINT('Ctrl Pts',(1.3735491215176,-0.237231147975234,-0.902193646979983));
#25002=CARTESIAN_POINT('Ctrl Pts',(1.36127834356734,-0.266264900654908,
-0.920778333482565));
#25003=CARTESIAN_POINT('Ctrl Pts',(1.33211611256184,-0.317195968905306,
-0.962485392528369));
#25004=CARTESIAN_POINT('Ctrl Pts',(1.31521005565926,-0.33909093068465,-0.985600426557816));
#25005=CARTESIAN_POINT('Ctrl Pts',(1.27866649102984,-0.373586846396559,
-1.03253285680459));
#25006=CARTESIAN_POINT('Ctrl Pts',(1.25722555095714,-0.388086240756494,
-1.05871835910697));
#25007=CARTESIAN_POINT('Ctrl Pts',(1.2107812086231,-0.407068917407805,-1.11153475808518));
#25008=CARTESIAN_POINT('Ctrl Pts',(1.18575674747573,-0.411552957311693,
-1.13814686046673));
#25009=CARTESIAN_POINT('Ctrl Pts',(1.13814686046673,-0.411552957311693,
-1.18575674747573));
#25010=CARTESIAN_POINT('Ctrl Pts',(1.11153475808518,-0.407068917407805,
-1.2107812086231));
#25011=CARTESIAN_POINT('Ctrl Pts',(1.05871835910697,-0.388086240756494,
-1.25722555095714));
#25012=CARTESIAN_POINT('Ctrl Pts',(1.03253285680459,-0.373586846396559,
-1.27866649102984));
#25013=CARTESIAN_POINT('Ctrl Pts',(0.985600426557816,-0.33909093068465,
-1.31521005565926));
#25014=CARTESIAN_POINT('Ctrl Pts',(0.962485392528369,-0.317195968905306,
-1.33211611256184));
#25015=CARTESIAN_POINT('Ctrl Pts',(0.920778333482565,-0.266264900654909,
-1.36127834356734));
#25016=CARTESIAN_POINT('Ctrl Pts',(0.902193646979983,-0.237231147975234,
-1.3735491215176));
#25017=CARTESIAN_POINT('Ctrl Pts',(0.867957148219442,-0.166543350814306,
-1.39550172959303));
#25018=CARTESIAN_POINT('Ctrl Pts',(0.854205272175555,-0.123401821157026,
-1.40380622184538));
#25019=CARTESIAN_POINT('Ctrl Pts',(0.846804978391753,-0.0793800000000001,
-1.40825612658882));
#25020=CARTESIAN_POINT('Origin',(1.18440385848747,-0.07938,-1.18440385848747));
#25021=CARTESIAN_POINT('Origin',(0.,-0.27783,0.));
#25022=CARTESIAN_POINT('',(-1.643248,-0.47628,2.01239840340529E-16));
#25023=CARTESIAN_POINT('Origin',(0.,-0.47628,0.));
#25024=CARTESIAN_POINT('',(-1.643248,-0.27783,2.01239840340529E-16));
#25025=CARTESIAN_POINT('',(1.59456899932179,-0.07938,0.397005914195118));
#25026=CARTESIAN_POINT('Origin',(0.,-0.07938,0.));
#25027=CARTESIAN_POINT('',(1.59456899932179,-0.07938,-0.397005914195118));
#25028=CARTESIAN_POINT('Ctrl Pts',(1.59456899932179,-0.0793800000000001,
0.397005914195118));
#25029=CARTESIAN_POINT('Ctrl Pts',(1.59665523941937,-0.123401821157026,
0.388626558458099));
#25030=CARTESIAN_POINT('Ctrl Pts',(1.60050712143809,-0.166543350814306,
0.373030350867485));
#25031=CARTESIAN_POINT('Ctrl Pts',(1.60919314384089,-0.237231147975234,
0.333298652394954));
#25032=CARTESIAN_POINT('Ctrl Pts',(1.61365775139403,-0.266264900654909,
0.311480544243686));
#25033=CARTESIAN_POINT('Ctrl Pts',(1.62252828437015,-0.317195968905306,
0.261368388670537));
#25034=CARTESIAN_POINT('Ctrl Pts',(1.62691869420078,-0.33909093068465,0.233069203882014));
#25035=CARTESIAN_POINT('Ctrl Pts',(1.63426473152765,-0.373586846396559,
0.174042761838764));
#25036=CARTESIAN_POINT('Ctrl Pts',(1.63761964365402,-0.388086240756494,
0.140365781471549));
#25037=CARTESIAN_POINT('Ctrl Pts',(1.64212536811722,-0.407068917407805,
0.0701778381840612));
#25038=CARTESIAN_POINT('Ctrl Pts',(1.643248,-0.411552957311693,0.0336652739555916));
#25039=CARTESIAN_POINT('Ctrl Pts',(1.643248,-0.411552957311693,-0.0336652739555916));
#25040=CARTESIAN_POINT('Ctrl Pts',(1.64212536811722,-0.407068917407805,
-0.0701778381840612));
#25041=CARTESIAN_POINT('Ctrl Pts',(1.63761964365402,-0.388086240756494,
-0.140365781471549));
#25042=CARTESIAN_POINT('Ctrl Pts',(1.63426473152765,-0.373586846396559,
-0.174042761838764));
#25043=CARTESIAN_POINT('Ctrl Pts',(1.62691869420078,-0.33909093068465,-0.233069203882014));
#25044=CARTESIAN_POINT('Ctrl Pts',(1.62252828437015,-0.317195968905306,
-0.261368388670537));
#25045=CARTESIAN_POINT('Ctrl Pts',(1.61365775139403,-0.266264900654909,
-0.311480544243686));
#25046=CARTESIAN_POINT('Ctrl Pts',(1.60919314384089,-0.237231147975234,
-0.333298652394954));
#25047=CARTESIAN_POINT('Ctrl Pts',(1.60050712143809,-0.166543350814306,
-0.373030350867485));
#25048=CARTESIAN_POINT('Ctrl Pts',(1.59665523941937,-0.123401821157026,
-0.388626558458099));
#25049=CARTESIAN_POINT('Ctrl Pts',(1.59456899932179,-0.07938,-0.397005914195118));
#25050=CARTESIAN_POINT('Origin',(0.,-0.07938,0.));
#25051=CARTESIAN_POINT('Origin',(0.,-0.07938,0.));
#25052=CARTESIAN_POINT('Origin',(1.675,-0.07938,0.));
#25053=CARTESIAN_POINT('Origin',(1.675,0.,0.));
#25054=CARTESIAN_POINT('Origin',(1.675,-0.07938,0.));
#25055=CARTESIAN_POINT('Origin',(0.,-0.47628,0.));
#25056=CARTESIAN_POINT('Origin',(0.,-0.07938,0.));
#62634=UNCERTAINTY_MEASURE_WITH_UNIT(LENGTH_MEASURE(0.001),#62759,
'DISTANCE_ACCURACY_VALUE',
'Maximum model space distance between geometric entities at asserted c
onnectivities');
#62684=UNCERTAINTY_MEASURE_WITH_UNIT(LENGTH_MEASURE(0.001),#62759,
'DISTANCE_ACCURACY_VALUE',
'Maximum model space distance between geometric entities at asserted c
onnectivities');
#62708=(
GEOMETRIC_REPRESENTATION_CONTEXT(3)
GLOBAL_UNCERTAINTY_ASSIGNED_CONTEXT((#62634))
GLOBAL_UNIT_ASSIGNED_CONTEXT((#62759,#62761,#62762))
REPRESENTATION_CONTEXT('','3D')
);
#62758=(
GEOMETRIC_REPRESENTATION_CONTEXT(3)
GLOBAL_UNCERTAINTY_ASSIGNED_CONTEXT((#62684))
GLOBAL_UNIT_ASSIGNED_CONTEXT((#62759,#62761,#62762))
REPRESENTATION_CONTEXT('','3D')
);
#62759=(
LENGTH_UNIT()
NAMED_UNIT(*)
SI_UNIT(.CENTI.,.METRE.)
);
#62761=(
NAMED_UNIT(*)
PLANE_ANGLE_UNIT()
SI_UNIT($,.RADIAN.)
);
#62762=(
NAMED_UNIT(*)
SI_UNIT($,.STERADIAN.)
SOLID_ANGLE_UNIT()
);
#62786=SHAPE_DEFINITION_REPRESENTATION(#62864,#63054);
#62864=PRODUCT_DEFINITION_SHAPE('',$,#63128);
#63054=SHAPE_REPRESENTATION('',(#17670),#62708);
#63104=PRODUCT_DEFINITION_CONTEXT('part definition',#63325,'design');
#63128=PRODUCT_DEFINITION('Cage (1)','Cage (1)',#63201,#63104);
#63201=PRODUCT_DEFINITION_FORMATION('',$,#63350);
#63325=APPLICATION_CONTEXT(
'Core Data for Automotive Mechanical Design Process');
#63326=PRODUCT_CONTEXT('part definition',#63325,'mechanical');
#63350=PRODUCT('Cage (1)','Cage (1)','Cage (1)',(#63326));
#63456=COLOUR_RGB('Grey',0.48,0.52,0.57);
#63457=FILL_AREA_STYLE_COLOUR('',#63456);
#63458=FILL_AREA_STYLE('',(#63457));
#63459=SURFACE_STYLE_FILL_AREA(#63458);
#63460=SURFACE_SIDE_STYLE('',(#63459));
#63461=SURFACE_STYLE_USAGE(.BOTH.,#63460);
#63462=PRESENTATION_STYLE_ASSIGNMENT((#63461));
ENDSEC;
END-ISO-10303-21;
